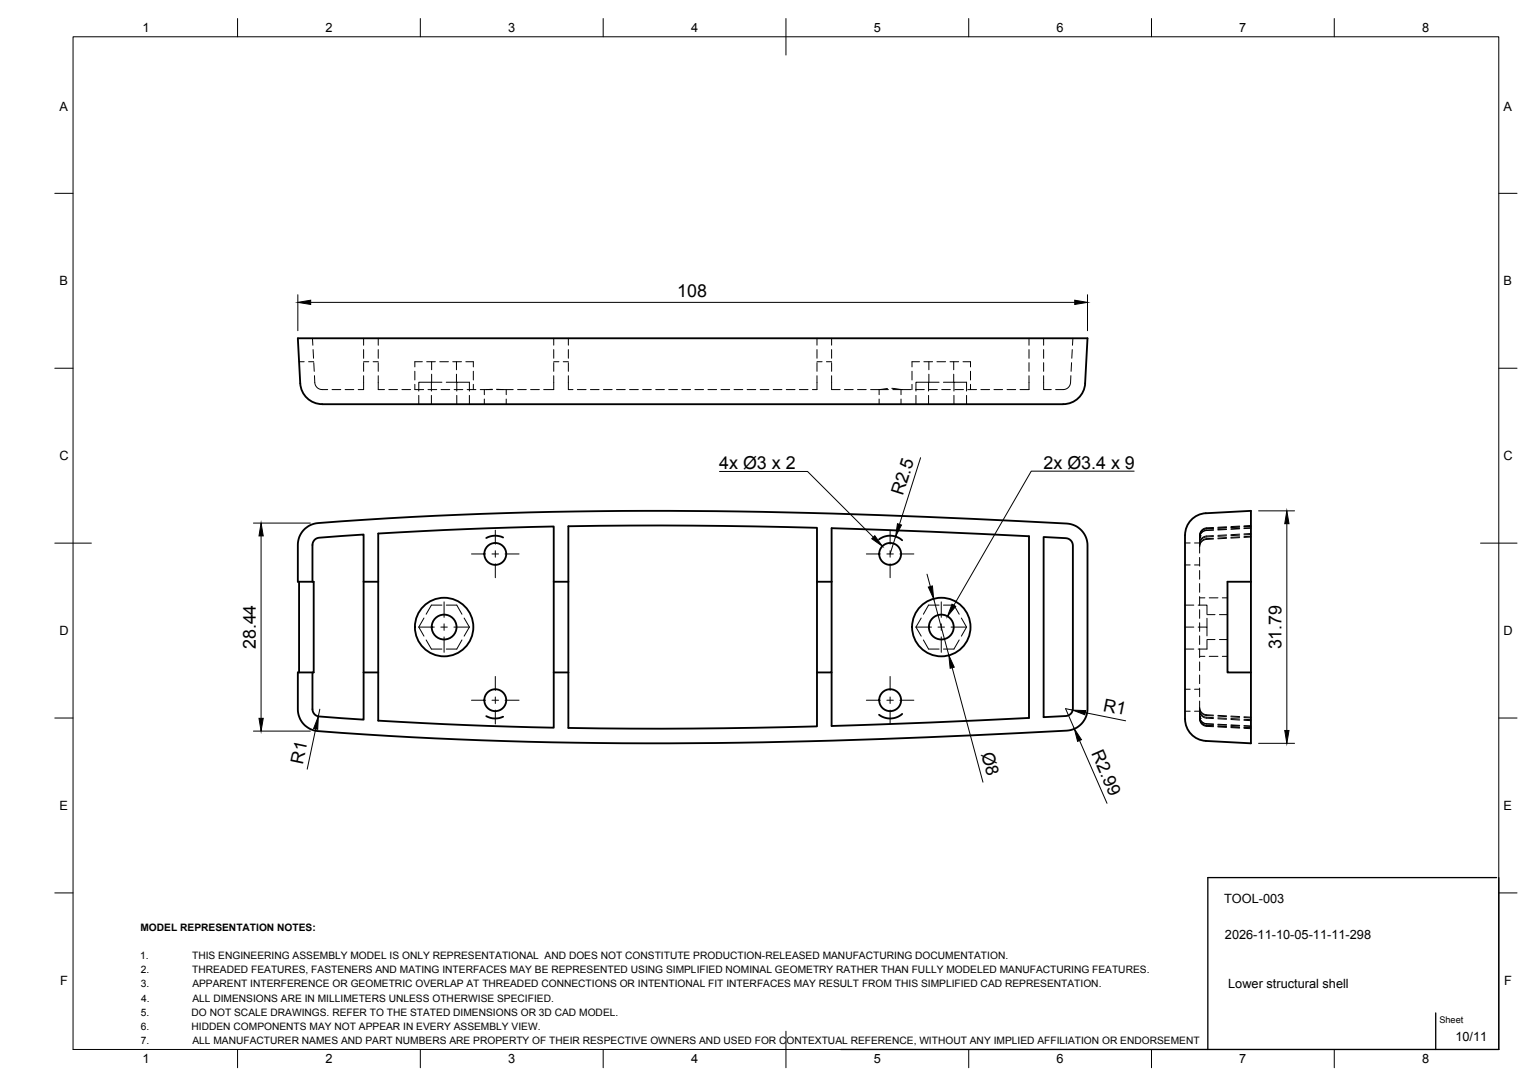
ISO-10303-21;
HEADER;
/* Generated by software containing ST-Developer
 * from STEP Tools, Inc. (www.steptools.com) 
 */

FILE_DESCRIPTION(
/* description */ (''),
/* implementation_level */ '2;1');

FILE_NAME(
/* name */ 'Lower structural shell.step',
/* time_stamp */ '2026-11-10T05:20:16-08:00',
/* author */ (''),
/* organization */ (''),
/* preprocessor_version */ 'ST-DEVELOPER v20.2',
/* originating_system */ 'Autodesk Translation Framework v15.17.0.0',
/* authorisation */ '');

FILE_SCHEMA (('AUTOMOTIVE_DESIGN { 1 0 10303 214 3 1 1 }'));
ENDSEC;

DATA;
#10=MECHANICAL_DESIGN_GEOMETRIC_PRESENTATION_REPRESENTATION('',(#117),#24809);
#84=SPHERICAL_SURFACE('',#10450,0.1);
#85=SPHERICAL_SURFACE('',#10453,0.0999999999999998);
#86=SPHERICAL_SURFACE('',#10457,0.0999999999999993);
#87=SPHERICAL_SURFACE('',#10461,0.1);
#88=SPHERICAL_SURFACE('',#10466,0.3);
#89=SPHERICAL_SURFACE('',#10470,0.3);
#90=SPHERICAL_SURFACE('',#10474,0.299999999999999);
#91=SPHERICAL_SURFACE('',#10479,0.3);
#97=SHAPE_REPRESENTATION_RELATIONSHIP('SRR','None',#24861,#107);
#107=ADVANCED_BREP_SHAPE_REPRESENTATION('',(#127),#24804);
#117=STYLED_ITEM('',(#24922),#127);
#127=MANIFOLD_SOLID_BREP('Body1',#9894);
#164=FACE_BOUND('',#2214,.T.);
#165=FACE_BOUND('',#2215,.T.);
#166=FACE_BOUND('',#2216,.T.);
#167=FACE_BOUND('',#2224,.T.);
#168=FACE_BOUND('',#2232,.T.);
#169=FACE_BOUND('',#2247,.T.);
#170=FACE_BOUND('',#2249,.T.);
#171=FACE_BOUND('',#2261,.T.);
#172=FACE_BOUND('',#2282,.T.);
#173=FACE_BOUND('',#2283,.T.);
#174=FACE_BOUND('',#2284,.T.);
#175=FACE_BOUND('',#2319,.T.);
#176=FACE_BOUND('',#2320,.T.);
#177=FACE_BOUND('',#2321,.T.);
#178=FACE_BOUND('',#2322,.T.);
#179=FACE_BOUND('',#2323,.T.);
#180=FACE_BOUND('',#2324,.T.);
#237=B_SPLINE_SURFACE_WITH_KNOTS('',3,3,((#17088,#17089,#17090,#17091),
(#17092,#17093,#17094,#17095),(#17096,#17097,#17098,#17099),(#17100,#17101,
#17102,#17103),(#17104,#17105,#17106,#17107)),.UNSPECIFIED.,.F.,.F.,.F.,
(4,1,4),(4,4),(0.,0.571428571428571,1.),(1.0454440030657,3.44967454744645),
 .UNSPECIFIED.);
#238=B_SPLINE_SURFACE_WITH_KNOTS('',3,3,((#17180,#17181,#17182,#17183),
(#17184,#17185,#17186,#17187),(#17188,#17189,#17190,#17191),(#17192,#17193,
#17194,#17195),(#17196,#17197,#17198,#17199)),.UNSPECIFIED.,.F.,.F.,.F.,
(4,1,4),(4,4),(0.,0.571428571428571,1.),(7.24519303641511,9.95046872158573),
 .UNSPECIFIED.);
#239=B_SPLINE_SURFACE_WITH_KNOTS('',3,3,((#18121,#18122,#18123,#18124),
(#18125,#18126,#18127,#18128),(#18129,#18130,#18131,#18132),(#18133,#18134,
#18135,#18136)),.UNSPECIFIED.,.F.,.F.,.F.,(4,4),(4,4),(0.0705535719740953,
0.323522444336189),(0.0117434863834119,0.684857763552191),.UNSPECIFIED.);
#240=B_SPLINE_SURFACE_WITH_KNOTS('',3,3,((#18141,#18142,#18143,#18144),
(#18145,#18146,#18147,#18148),(#18149,#18150,#18151,#18152),(#18153,#18154,
#18155,#18156)),.UNSPECIFIED.,.F.,.F.,.F.,(4,4),(4,4),(0.0262419052680539,
0.0545428296147404),(0.0121538053864343,0.684980602226481),
 .UNSPECIFIED.);
#241=B_SPLINE_SURFACE_WITH_KNOTS('',3,3,((#18166,#18167,#18168,#18169),
(#18170,#18171,#18172,#18173),(#18174,#18175,#18176,#18177),(#18178,#18179,
#18180,#18181),(#18182,#18183,#18184,#18185)),.UNSPECIFIED.,.F.,.F.,.F.,
(4,1,4),(4,4),(0.,0.571428571428571,1.),(0.752061768057538,3.45733745322815),
 .UNSPECIFIED.);
#242=B_SPLINE_SURFACE_WITH_KNOTS('',3,3,((#18186,#18187,#18188,#18189),
(#18190,#18191,#18192,#18193),(#18194,#18195,#18196,#18197),(#18198,#18199,
#18200,#18201),(#18202,#18203,#18204,#18205)),.UNSPECIFIED.,.F.,.F.,.F.,
(4,1,4),(4,4),(0.,0.571428571428571,1.),(0.283259008618247,0.557056952888827),
 .UNSPECIFIED.);
#243=B_SPLINE_SURFACE_WITH_KNOTS('',3,3,((#18219,#18220,#18221,#18222),
(#18223,#18224,#18225,#18226),(#18227,#18228,#18229,#18230),(#18231,#18232,
#18233,#18234)),.UNSPECIFIED.,.F.,.F.,.F.,(4,4),(4,4),(0.67647755566375,
0.929446428026011),(0.0117434863436937,0.684857763580381),.UNSPECIFIED.);
#244=B_SPLINE_SURFACE_WITH_KNOTS('',3,3,((#18235,#18236,#18237,#18238),
(#18239,#18240,#18241,#18242),(#18243,#18244,#18245,#18246),(#18247,#18248,
#18249,#18250)),.UNSPECIFIED.,.F.,.F.,.F.,(4,4),(4,4),(0.945457170385156,
0.973758094731946),(0.0121538053598088,0.684980602226481),.UNSPECIFIED.);
#245=B_SPLINE_SURFACE_WITH_KNOTS('',3,3,((#18334,#18335,#18336,#18337),
(#18338,#18339,#18340,#18341),(#18342,#18343,#18344,#18345),(#18346,#18347,
#18348,#18349)),.UNSPECIFIED.,.F.,.F.,.F.,(4,4),(4,4),(0.341142793678372,
0.658675488550287),(0.0116221239297273,0.684255166525269),.UNSPECIFIED.);
#246=B_SPLINE_SURFACE_WITH_KNOTS('',3,3,((#18354,#18355,#18356,#18357),
(#18358,#18359,#18360,#18361),(#18362,#18363,#18364,#18365),(#18366,#18367,
#18368,#18369),(#18370,#18371,#18372,#18373)),.UNSPECIFIED.,.F.,.F.,.F.,
(4,1,4),(4,4),(0.,0.571428571428571,1.),(3.65450559744172,7.0548588409572),
 .UNSPECIFIED.);
#247=B_SPLINE_SURFACE_WITH_KNOTS('',3,3,((#18383,#18384,#18385,#18386),
(#18387,#18388,#18389,#18390),(#18391,#18392,#18393,#18394),(#18395,#18396,
#18397,#18398),(#18399,#18400,#18401,#18402)),.UNSPECIFIED.,.F.,.F.,.F.,
(4,1,4),(4,4),(0.,0.571428571428571,1.),(3.64767164868607,7.04802489220155),
 .UNSPECIFIED.);
#248=B_SPLINE_SURFACE_WITH_KNOTS('',3,3,((#18407,#18408,#18409,#18410),
(#18411,#18412,#18413,#18414),(#18415,#18416,#18417,#18418),(#18419,#18420,
#18421,#18422)),.UNSPECIFIED.,.F.,.F.,.F.,(4,4),(4,4),(0.341324511449716,
0.658857206321627),(0.0116221214776208,0.684255166525269),.UNSPECIFIED.);
#249=B_SPLINE_SURFACE_WITH_KNOTS('',3,3,((#18467,#18468,#18469,#18470),
(#18471,#18472,#18473,#18474),(#18475,#18476,#18477,#18478),(#18479,#18480,
#18481,#18482)),.UNSPECIFIED.,.F.,.F.,.F.,(4,4),(4,4),(0.676316266718331,
0.901708040522105),(0.0117102006467275,0.68495201331719),.UNSPECIFIED.);
#250=B_SPLINE_SURFACE_WITH_KNOTS('',3,3,((#18487,#18488,#18489,#18490),
(#18491,#18492,#18493,#18494),(#18495,#18496,#18497,#18498),(#18499,#18500,
#18501,#18502),(#18503,#18504,#18505,#18506)),.UNSPECIFIED.,.F.,.F.,.F.,
(4,1,4),(4,4),(0.,0.571428571428571,1.),(7.25285594219682,9.65708648657758),
 .UNSPECIFIED.);
#251=B_SPLINE_SURFACE_WITH_KNOTS('',3,3,((#18516,#18517,#18518,#18519),
(#18520,#18521,#18522,#18523),(#18524,#18525,#18526,#18527),(#18528,#18529,
#18530,#18531)),.UNSPECIFIED.,.F.,.F.,.F.,(4,4),(4,4),(0.0982919594778951,
0.323683733281714),(0.0117102006467272,0.68495201331719),.UNSPECIFIED.);
#252=B_SPLINE_SURFACE_WITH_KNOTS('',3,3,((#18606,#18607,#18608,#18609),
(#18610,#18611,#18612,#18613),(#18614,#18615,#18616,#18617),(#18618,#18619,
#18620,#18621)),.UNSPECIFIED.,.F.,.F.,.F.,(4,4),(4,4),(0.917922863855343,
0.974411608827007),(0.0122403473423911,0.685344304754238),.UNSPECIFIED.);
#253=B_SPLINE_SURFACE_WITH_KNOTS('',3,3,((#18631,#18632,#18633,#18634),
(#18635,#18636,#18637,#18638),(#18639,#18640,#18641,#18642),(#18643,#18644,
#18645,#18646),(#18647,#18648,#18649,#18650)),.UNSPECIFIED.,.F.,.F.,.F.,
(4,1,4),(4,4),(0.,0.571428571428571,1.),(9.85085636625011,10.4271318523291),
 .UNSPECIFIED.);
#254=B_SPLINE_SURFACE_WITH_KNOTS('',3,3,((#18664,#18665,#18666,#18667),
(#18668,#18669,#18670,#18671),(#18672,#18673,#18674,#18675),(#18676,#18677,
#18678,#18679)),.UNSPECIFIED.,.F.,.F.,.F.,(4,4),(4,4),(0.025588391172993,
0.0820771361446569),(0.0122403473423911,0.685344304754238),
 .UNSPECIFIED.);
#255=B_SPLINE_SURFACE_WITH_KNOTS('',3,3,((#18689,#18690,#18691,#18692),
(#18693,#18694,#18695,#18696),(#18697,#18698,#18699,#18700),(#18701,#18702,
#18703,#18704),(#18705,#18706,#18707,#18708)),.UNSPECIFIED.,.F.,.F.,.F.,
(4,1,4),(4,4),(0.,0.571428571428571,1.),(0.27539863731415,0.851674123393175),
 .UNSPECIFIED.);
#256=B_SPLINE_SURFACE_WITH_KNOTS('',3,3,((#18722,#18723,#18724,#18725),
(#18726,#18727,#18728,#18729),(#18730,#18731,#18732,#18733),(#18734,#18735,
#18736,#18737),(#18738,#18739,#18740,#18741)),.UNSPECIFIED.,.F.,.F.,.F.,
(4,1,4),(4,4),(0.,0.571428571428571,1.),(0.00944995813270487,0.618489359031386),
 .UNSPECIFIED.);
#257=B_SPLINE_SURFACE_WITH_KNOTS('',3,3,((#18748,#18749,#18750,#18751),
(#18752,#18753,#18754,#18755),(#18756,#18757,#18758,#18759),(#18760,#18761,
#18762,#18763),(#18764,#18765,#18766,#18767)),.UNSPECIFIED.,.F.,.F.,.F.,
(4,1,4),(4,4),(0.,0.571428571428571,1.),(0.00908570715245136,0.618164468641375),
 .UNSPECIFIED.);
#258=B_SPLINE_SURFACE_WITH_KNOTS('',3,3,((#18772,#18773,#18774,#18775),
(#18776,#18777,#18778,#18779),(#18780,#18781,#18782,#18783),(#18784,#18785,
#18786,#18787),(#18788,#18789,#18790,#18791)),.UNSPECIFIED.,.F.,.F.,.F.,
(4,1,4),(4,4),(0.,0.571428571428571,1.),(0.0091183540525243,0.618164468641375),
 .UNSPECIFIED.);
#259=B_SPLINE_SURFACE_WITH_KNOTS('',3,3,((#18796,#18797,#18798,#18799),
(#18800,#18801,#18802,#18803),(#18804,#18805,#18806,#18807),(#18808,#18809,
#18810,#18811),(#18812,#18813,#18814,#18815)),.UNSPECIFIED.,.F.,.F.,.F.,
(4,1,4),(4,4),(0.,0.571428571428571,1.),(10.1454735367545,10.419271481025),
 .UNSPECIFIED.);
#260=B_SPLINE_SURFACE_WITH_KNOTS('',3,3,((#18816,#18817,#18818,#18819),
(#18820,#18821,#18822,#18823),(#18824,#18825,#18826,#18827),(#18828,#18829,
#18830,#18831),(#18832,#18833,#18834,#18835)),.UNSPECIFIED.,.F.,.F.,.F.,
(4,1,4),(4,4),(0.,0.571428571428571,1.),(0.0094045468285345,0.618489359031386),
 .UNSPECIFIED.);
#261=B_SPLINE_SURFACE_WITH_KNOTS('',3,3,((#18861,#18862,#18863,#18864),
(#18865,#18866,#18867,#18868),(#18869,#18870,#18871,#18872),(#18873,#18874,
#18875,#18876),(#18877,#18878,#18879,#18880)),.UNSPECIFIED.,.F.,.F.,.F.,
(4,1,4),(4,4),(0.,0.571428571428571,1.),(-0.00535061636073277,0.618489359031386),
 .UNSPECIFIED.);
#262=B_SPLINE_SURFACE_WITH_KNOTS('',3,3,((#18899,#18900,#18901,#18902,#18903),
(#18904,#18905,#18906,#18907,#18908),(#18909,#18910,#18911,#18912,#18913),
(#18914,#18915,#18916,#18917,#18918),(#18919,#18920,#18921,#18922,#18923)),
 .UNSPECIFIED.,.F.,.F.,.F.,(4,1,4),(4,1,4),(0.,0.571428571428571,1.),(0.283259008618247,
4.63063308449434,10.4271318523291),.UNSPECIFIED.);
#263=B_SPLINE_SURFACE_WITH_KNOTS('',3,3,((#18934,#18935,#18936,#18937),
(#18938,#18939,#18940,#18941),(#18942,#18943,#18944,#18945),(#18946,#18947,
#18948,#18949),(#18950,#18951,#18952,#18953)),.UNSPECIFIED.,.F.,.F.,.F.,
(4,1,4),(4,4),(0.,0.571428571428571,1.),(-0.00578978989683084,0.618164468641375),
 .UNSPECIFIED.);
#264=B_SPLINE_SURFACE_WITH_KNOTS('',3,3,((#18962,#18963,#18964,#18965),
(#18966,#18967,#18968,#18969),(#18970,#18971,#18972,#18973),(#18974,#18975,
#18976,#18977),(#18978,#18979,#18980,#18981)),.UNSPECIFIED.,.F.,.F.,.F.,
(4,1,4),(4,4),(0.,0.571428571428571,1.),(-0.00569189159989896,0.618164468641375),
 .UNSPECIFIED.);
#265=B_SPLINE_SURFACE_WITH_KNOTS('',3,3,((#18990,#18991,#18992,#18993,#18994),
(#18995,#18996,#18997,#18998,#18999),(#19000,#19001,#19002,#19003,#19004),
(#19005,#19006,#19007,#19008,#19009),(#19010,#19011,#19012,#19013,#19014)),
 .UNSPECIFIED.,.F.,.F.,.F.,(4,1,4),(4,1,4),(0.,0.571428571428571,1.),(0.27539863731415,
4.62277271319024,10.419271481025),.UNSPECIFIED.);
#266=B_SPLINE_SURFACE_WITH_KNOTS('',3,3,((#19025,#19026,#19027,#19028),
(#19029,#19030,#19031,#19032),(#19033,#19034,#19035,#19036),(#19037,#19038,
#19039,#19040),(#19041,#19042,#19043,#19044)),.UNSPECIFIED.,.F.,.F.,.F.,
(4,1,4),(4,4),(0.,0.571428571428571,1.),(-0.0054868135546625,0.618489359031386),
 .UNSPECIFIED.);
#267=B_SPLINE_SURFACE_WITH_KNOTS('',3,3,((#19053,#19054,#19055,#19056),
(#19057,#19058,#19059,#19060),(#19061,#19062,#19063,#19064),(#19065,#19066,
#19067,#19068)),.UNSPECIFIED.,.F.,.F.,.F.,(4,4),(4,4),(0.026239262514127,
0.974414173651419),(0.,0.685344304754238),.UNSPECIFIED.);
#268=B_SPLINE_SURFACE_WITH_KNOTS('',3,3,((#19071,#19072,#19073,#19074),
(#19075,#19076,#19077,#19078),(#19079,#19080,#19081,#19082),(#19083,#19084,
#19085,#19086)),.UNSPECIFIED.,.F.,.F.,.F.,(4,4),(4,4),(0.0255858263485814,
0.973760737485873),(0.,0.685344304754238),.UNSPECIFIED.);
#717=B_SPLINE_CURVE_WITH_KNOTS('',3,(#16987,#16988,#16989,#16990,#16991,
#16992,#16993,#16994,#16995,#16996,#16997,#16998,#16999,#17000,#17001,#17002,
#17003,#17004,#17005,#17006,#17007,#17008,#17009,#17010),.UNSPECIFIED.,
 .F.,.F.,(4,2,2,2,2,2,2,2,2,2,2,4),(-0.337265338267783,-0.250544943628509,
-0.208272806508042,-0.186542211788094,-0.176382978682897,-0.170925844043069,
-0.16639450677335,-0.161077381235501,-0.15182241135393,-0.115009181549223,
-0.030206004227969,0.),.UNSPECIFIED.);
#718=B_SPLINE_CURVE_WITH_KNOTS('',3,(#17015,#17016,#17017,#17018,#17019,
#17020,#17021,#17022,#17023,#17024,#17025,#17026,#17027,#17028,#17029,#17030,
#17031,#17032,#17033,#17034),.UNSPECIFIED.,.F.,.F.,(4,2,2,2,2,2,2,2,2,4),
(-0.240982594686416,-0.16829976149504,-0.141836598208813,-0.129116059226128,
-0.121962912034391,-0.115857591426886,-0.108506552485159,-0.0948769875819265,
-0.0364654790774683,0.),.UNSPECIFIED.);
#719=B_SPLINE_CURVE_WITH_KNOTS('',3,(#17039,#17040,#17041,#17042,#17043,
#17044,#17045,#17046,#17047,#17048,#17049,#17050,#17051,#17052,#17053,#17054,
#17055,#17056,#17057,#17058),.UNSPECIFIED.,.F.,.F.,(4,2,2,2,2,2,2,2,2,4),
(-0.240981214998207,-0.168303541671295,-0.141841407502325,-0.129121097580905,
-0.121968013294536,-0.115862708924237,-0.108511643765797,-0.0948818976588229,
-0.0364681276985956,0.),.UNSPECIFIED.);
#720=B_SPLINE_CURVE_WITH_KNOTS('',3,(#17063,#17064,#17065,#17066,#17067,
#17068,#17069,#17070,#17071,#17072,#17073,#17074,#17075,#17076,#17077,#17078,
#17079,#17080,#17081,#17082,#17083,#17084,#17085,#17086),.UNSPECIFIED.,
 .F.,.F.,(4,2,2,2,2,2,2,2,2,2,2,4),(-0.337269388373684,-0.250545316912909,
-0.208282401844766,-0.186554569827561,-0.176396213396297,-0.17093921790305,
-0.16640782243471,-0.161090427650893,-0.151834477986603,-0.115010808423941,
-0.0302102096065556,0.),.UNSPECIFIED.);
#721=B_SPLINE_CURVE_WITH_KNOTS('',3,(#17109,#17110,#17111,#17112),
 .UNSPECIFIED.,.F.,.F.,(4,4),(1.0454440030657,2.52465537163019),
 .UNSPECIFIED.);
#722=B_SPLINE_CURVE_WITH_KNOTS('',3,(#17114,#17115,#17116,#17117,#17118,
#17119,#17120,#17121,#17122,#17123,#17124,#17125,#17126,#17127,#17128,#17129,
#17130,#17131,#17132,#17133,#17134,#17135,#17136,#17137,#17138,#17139,#17140,
#17141),.UNSPECIFIED.,.F.,.F.,(4,3,3,3,3,3,3,3,3,4),(-0.152193408756968,
-0.128427023368412,-0.115107736263918,-0.0911810900745799,-0.0780377802127556,
-0.0652031397886901,-0.0414031558437525,-0.0389949527774582,-0.0152076153333754,
0.),.UNSPECIFIED.);
#723=B_SPLINE_CURVE_WITH_KNOTS('',3,(#17143,#17144,#17145,#17146),
 .UNSPECIFIED.,.F.,.F.,(4,4),(-3.44967454744645,-1.05170160817356),
 .UNSPECIFIED.);
#724=B_SPLINE_CURVE_WITH_KNOTS('',3,(#17148,#17149,#17150,#17151,#17152,
#17153,#17154,#17155,#17156,#17157,#17158,#17159,#17160,#17161,#17162,#17163,
#17164,#17165,#17166,#17167,#17168,#17169,#17170,#17171,#17172,#17173,#17174,
#17175),.UNSPECIFIED.,.F.,.F.,(4,3,3,3,3,3,3,3,3,4),(-0.152278960443096,
-0.128503570101575,-0.115218572146868,-0.09145408274965,-0.0870214650669139,
-0.0781562978024333,-0.0542566895399357,-0.03908030849237,-0.0153296112319379,
0.),.UNSPECIFIED.);
#725=B_SPLINE_CURVE_WITH_KNOTS('',3,(#17176,#17177,#17178,#17179),
 .UNSPECIFIED.,.F.,.F.,(4,4),(2.75501813708031,3.4476340663212),
 .UNSPECIFIED.);
#726=B_SPLINE_CURVE_WITH_KNOTS('',3,(#17201,#17202,#17203,#17204),
 .UNSPECIFIED.,.F.,.F.,(4,4),(7.24810383506675,7.89761558728778),
 .UNSPECIFIED.);
#727=B_SPLINE_CURVE_WITH_KNOTS('',3,(#17206,#17207,#17208,#17209,#17210,
#17211,#17212,#17213,#17214,#17215,#17216,#17217,#17218,#17219,#17220,#17221,
#17222,#17223,#17224,#17225,#17226,#17227,#17228,#17229,#17230,#17231,#17232,
#17233),.UNSPECIFIED.,.F.,.F.,(4,3,3,3,3,3,3,3,3,4),(-0.152278869104567,
-0.128548794904564,-0.115192257893812,-0.0912773536606376,-0.0781090575823055,
-0.0652724057916263,-0.0414819581560496,-0.0390493575290778,-0.015259721743698,
0.),.UNSPECIFIED.);
#728=B_SPLINE_CURVE_WITH_KNOTS('',3,(#17235,#17236,#17237,#17238),
 .UNSPECIFIED.,.F.,.F.,(4,4),(-9.94532343034734,-7.24519303641511),
 .UNSPECIFIED.);
#729=B_SPLINE_CURVE_WITH_KNOTS('',3,(#17240,#17241,#17242,#17243,#17244,
#17245,#17246,#17247,#17248,#17249,#17250,#17251,#17252,#17253,#17254,#17255,
#17256,#17257,#17258,#17259,#17260,#17261,#17262,#17263,#17264,#17265,#17266,
#17267),.UNSPECIFIED.,.F.,.F.,(4,3,3,3,3,3,3,3,3,4),(-0.152181623618259,
-0.128410404494075,-0.115248188224843,-0.0914746846046984,-0.0869904866333268,
-0.0783028696190655,-0.0543945376065823,-0.0391651209697638,-0.0153884182770307,
0.),.UNSPECIFIED.);
#730=B_SPLINE_CURVE_WITH_KNOTS('',3,(#17268,#17269,#17270,#17271),
 .UNSPECIFIED.,.F.,.F.,(4,4),(8.21380824320284,9.95046871680089),
 .UNSPECIFIED.);
#731=B_SPLINE_CURVE_WITH_KNOTS('',3,(#17274,#17275,#17276,#17277),
 .UNSPECIFIED.,.F.,.F.,(4,4),(2.80491490332713,3.45442665446657),
 .UNSPECIFIED.);
#732=B_SPLINE_CURVE_WITH_KNOTS('',3,(#17281,#17282,#17283,#17284),
 .UNSPECIFIED.,.F.,.F.,(4,4),(0.752061768057538,2.48872224644044),
 .UNSPECIFIED.);
#733=B_SPLINE_CURVE_WITH_KNOTS('',3,(#17492,#17493,#17494,#17495,#17496,
#17497),.UNSPECIFIED.,.F.,.F.,(4,2,4),(-0.606700505977711,-0.303383635264422,
-0.000339350725729326),.UNSPECIFIED.);
#734=B_SPLINE_CURVE_WITH_KNOTS('',3,(#17498,#17499,#17500,#17501,#17502,
#17503,#17504,#17505,#17506,#17507,#17508,#17509,#17510,#17511,#17512,#17513,
#17514,#17515,#17516,#17517,#17518,#17519,#17520,#17521,#17522,#17523,#17524,
#17525),.UNSPECIFIED.,.F.,.F.,(4,3,3,3,3,3,3,3,3,4),(-0.152173579228948,
-0.128423230539522,-0.115115104157663,-0.0911927259648815,-0.0780672068328041,
-0.0652082609452843,-0.0414117413801899,-0.0390174000215468,-0.0152300060615686,
0.),.UNSPECIFIED.);
#735=B_SPLINE_CURVE_WITH_KNOTS('',3,(#17526,#17527,#17528,#17529,#17530,
#17531),.UNSPECIFIED.,.F.,.F.,(4,2,4),(-0.606471894652381,-0.303383500305553,
-0.00011071898471493),.UNSPECIFIED.);
#736=B_SPLINE_CURVE_WITH_KNOTS('',3,(#17535,#17536,#17537,#17538,#17539,
#17540),.UNSPECIFIED.,.F.,.F.,(4,2,4),(-0.606240625011114,-0.303433113375332,
-0.00010938105916114),.UNSPECIFIED.);
#737=B_SPLINE_CURVE_WITH_KNOTS('',3,(#17542,#17543,#17544,#17545,#17546,
#17547,#17548,#17549,#17550,#17551,#17552,#17553,#17554,#17555,#17556,#17557,
#17558,#17559,#17560,#17561,#17562,#17563,#17564,#17565,#17566,#17567,#17568,
#17569),.UNSPECIFIED.,.F.,.F.,(4,3,3,3,3,3,3,3,3,4),(-0.152281454644235,
-0.128508102092242,-0.115234945630277,-0.0914677943501604,-0.0870276017853555,
-0.0781846052914712,-0.0542821334115454,-0.0390966859411886,-0.0153419673568312,
0.),.UNSPECIFIED.);
#738=B_SPLINE_CURVE_WITH_KNOTS('',3,(#17571,#17572,#17573,#17574,#17575,
#17576),.UNSPECIFIED.,.F.,.F.,(4,2,4),(-0.606758573154242,-0.303433157101101,
-0.000627306481538803),.UNSPECIFIED.);
#739=B_SPLINE_CURVE_WITH_KNOTS('',3,(#17582,#17583,#17584,#17585,#17586,
#17587),.UNSPECIFIED.,.F.,.F.,(4,2,4),(-0.60617382748,-0.303436117212405,
-7.2700296824213E-5),.UNSPECIFIED.);
#740=B_SPLINE_CURVE_WITH_KNOTS('',3,(#17589,#17590,#17591,#17592,#17593,
#17594,#17595,#17596,#17597,#17598,#17599,#17600,#17601,#17602,#17603,#17604,
#17605,#17606,#17607,#17608,#17609,#17610,#17611,#17612,#17613,#17614,#17615,
#17616),.UNSPECIFIED.,.F.,.F.,(4,3,3,3,3,3,3,3,3,4),(-0.152282154327755,
-0.128558036203745,-0.115201429639692,-0.0912891813973639,-0.0781219052297615,
-0.065279687589213,-0.0414913146723999,-0.0390591331507366,-0.0152683745546824,
0.),.UNSPECIFIED.);
#741=B_SPLINE_CURVE_WITH_KNOTS('',3,(#17620,#17621,#17622,#17623,#17624,
#17625,#17626,#17627,#17628,#17629,#17630,#17631,#17632,#17633,#17634,#17635,
#17636,#17637,#17638,#17639,#17640,#17641,#17642,#17643,#17644,#17645,#17646,
#17647),.UNSPECIFIED.,.F.,.F.,(4,3,3,3,3,3,3,3,3,4),(-0.152283066055976,
-0.128508717930245,-0.115216472798554,-0.091451700383826,-0.087022506454752,
-0.0781485278686168,-0.0542483994686567,-0.0390758108455304,-0.0153274175274101,
0.),.UNSPECIFIED.);
#742=B_SPLINE_CURVE_WITH_KNOTS('',3,(#17649,#17650,#17651,#17652,#17653,
#17654),.UNSPECIFIED.,.F.,.F.,(4,2,4),(-0.606800264911061,-0.303436147592132,
-0.000699137727853738),.UNSPECIFIED.);
#743=B_SPLINE_CURVE_WITH_KNOTS('',3,(#17659,#17660,#17661,#17662,#17663,
#17664),.UNSPECIFIED.,.F.,.F.,(4,2,4),(-0.606915279655722,-0.30363236403835,
-0.000516487074480598),.UNSPECIFIED.);
#744=B_SPLINE_CURVE_WITH_KNOTS('',3,(#17668,#17669,#17670,#17671,#17672,
#17673,#17674,#17675,#17676,#17677,#17678,#17679,#17680,#17681,#17682,#17683,
#17684,#17685,#17686,#17687,#17688,#17689,#17690,#17691,#17692,#17693,#17694,
#17695),.UNSPECIFIED.,.F.,.F.,(4,3,3,3,3,3,3,3,3,4),(-0.152205325335401,
-0.128433618138404,-0.115304790388008,-0.091527299141506,-0.0870178586418932,
-0.0783866443643876,-0.0544751548276533,-0.0392137310602028,-0.0154203878854647,
0.),.UNSPECIFIED.);
#745=B_SPLINE_CURVE_WITH_KNOTS('',3,(#17697,#17698,#17699,#17700,#17701,
#17702),.UNSPECIFIED.,.F.,.F.,(4,2,4),(-0.606752424187958,-0.303632696349781,
-0.000353591088346872),.UNSPECIFIED.);
#746=B_SPLINE_CURVE_WITH_KNOTS('',3,(#17708,#17709,#17710,#17711),
 .UNSPECIFIED.,.F.,.F.,(4,4),(0.0116023361771303,0.618489359031386),
 .UNSPECIFIED.);
#747=B_SPLINE_CURVE_WITH_KNOTS('',3,(#17715,#17716,#17717,#17718),
 .UNSPECIFIED.,.F.,.F.,(4,4),(-0.618489359031386,-0.01160233617713),
 .UNSPECIFIED.);
#748=B_SPLINE_CURVE_WITH_KNOTS('',3,(#17721,#17722,#17723,#17724),
 .UNSPECIFIED.,.F.,.F.,(4,4),(7.01593971618694,9.71770560667459),
 .UNSPECIFIED.);
#749=B_SPLINE_CURVE_WITH_KNOTS('',3,(#17725,#17726,#17727,#17728),
 .UNSPECIFIED.,.F.,.F.,(4,4),(0.505945342046796,3.20718651982575),
 .UNSPECIFIED.);
#750=B_SPLINE_CURVE_WITH_KNOTS('',3,(#17731,#17732,#17733,#17734,#17735,
#17736,#17737),.UNSPECIFIED.,.F.,.F.,(4,3,4),(3.40717417387402,5.11170895874517,
6.80746068626633),.UNSPECIFIED.);
#751=B_SPLINE_CURVE_WITH_KNOTS('',3,(#17740,#17741,#17742,#17743),
 .UNSPECIFIED.,.F.,.F.,(4,4),(7.00766573366377,9.41198845520559),
 .UNSPECIFIED.);
#752=B_SPLINE_CURVE_WITH_KNOTS('',3,(#17747,#17748,#17749,#17750),
 .UNSPECIFIED.,.F.,.F.,(4,4),(9.61248784142317,10.2217363065808),
 .UNSPECIFIED.);
#753=B_SPLINE_CURVE_WITH_KNOTS('',3,(#17751,#17752,#17753,#17754,#17755,
#17756,#17757,#17758,#17759,#17760,#17761,#17762,#17763,#17764,#17765,#17766,
#17767,#17768,#17769,#17770,#17771,#17772,#17773,#17774,#17775,#17776,#17777,
#17778),.UNSPECIFIED.,.F.,.F.,(4,3,3,3,3,3,3,3,3,4),(0.,0.0238103109064959,
0.0390781362249314,0.0628635086275546,0.0641230352384255,0.0780643700703951,
0.101962174814111,0.113803522271848,0.137549611554782,0.149564734365165),
 .UNSPECIFIED.);
#754=B_SPLINE_CURVE_WITH_KNOTS('',3,(#17782,#17783,#17784,#17785,#17786,
#17787,#17788,#17789,#17790,#17791,#17792,#17793,#17794,#17795,#17796,#17797,
#17798,#17799,#17800,#17801,#17802,#17803,#17804,#17805,#17806,#17807,#17808,
#17809,#17810,#17811,#17812),.UNSPECIFIED.,.F.,.F.,(4,3,3,3,3,3,3,3,3,3,
4),(0.,0.0535521515156599,0.107729685495911,0.117233338918226,0.171447998942947,
0.1923696899792,0.234191611538245,0.288659693466396,0.341410301570312,0.395549383747909,
0.448696573746633),.UNSPECIFIED.);
#755=B_SPLINE_CURVE_WITH_KNOTS('',3,(#17814,#17815,#17816,#17817),
 .UNSPECIFIED.,.F.,.F.,(4,4),(0.0255858263485814,0.973760737485873),
 .UNSPECIFIED.);
#756=B_SPLINE_CURVE_WITH_KNOTS('',3,(#17819,#17820,#17821,#17822,#17823,
#17824,#17825,#17826,#17827,#17828,#17829,#17830,#17831,#17832,#17833,#17834,
#17835,#17836,#17837,#17838,#17839,#17840,#17841,#17842,#17843,#17844,#17845,
#17846,#17847,#17848,#17849),.UNSPECIFIED.,.F.,.F.,(4,3,3,3,3,3,3,3,3,3,
4),(0.,0.0535144560117858,0.107726856902975,0.117300577410231,0.171517675930231,
0.195438847090422,0.234297456941738,0.289665153342662,0.345032849743585,
0.40043206955427,0.455831289364955),.UNSPECIFIED.);
#757=B_SPLINE_CURVE_WITH_KNOTS('',3,(#17853,#17854,#17855,#17856,#17857,
#17858,#17859,#17860,#17861,#17862,#17863,#17864,#17865,#17866,#17867,#17868,
#17869,#17870,#17871,#17872,#17873,#17874,#17875,#17876,#17877,#17878,#17879,
#17880,#17881,#17882,#17883),.UNSPECIFIED.,.F.,.F.,(4,3,3,3,3,3,3,3,3,3,
4),(0.,0.053505543180391,0.107714168832353,0.117253997025819,0.171473395203321,
0.195418854185489,0.234223199196375,0.289607016015183,0.344990832833991,
0.400409777473312,0.455828722112633),.UNSPECIFIED.);
#758=B_SPLINE_CURVE_WITH_KNOTS('',3,(#17885,#17886,#17887,#17888),
 .UNSPECIFIED.,.F.,.F.,(4,4),(0.0262392625141271,0.974414173651419),
 .UNSPECIFIED.);
#759=B_SPLINE_CURVE_WITH_KNOTS('',3,(#17890,#17891,#17892,#17893,#17894,
#17895,#17896,#17897,#17898,#17899,#17900,#17901,#17902,#17903,#17904,#17905,
#17906,#17907,#17908,#17909,#17910,#17911,#17912,#17913,#17914,#17915,#17916,
#17917,#17918,#17919,#17920),.UNSPECIFIED.,.F.,.F.,(4,3,3,3,3,3,3,3,3,3,
4),(0.,0.0535648734523888,0.107747221190676,0.117299947751206,0.171510987106922,
0.192397607227928,0.234296687348373,0.288768001369001,0.341469499352622,
0.395597672314973,0.448700135162036),.UNSPECIFIED.);
#760=B_SPLINE_CURVE_WITH_KNOTS('',3,(#17923,#17924,#17925,#17926,#17927,
#17928,#17929,#17930,#17931,#17932,#17933,#17934,#17935,#17936,#17937,#17938,
#17939,#17940,#17941,#17942,#17943,#17944,#17945,#17946,#17947),
 .UNSPECIFIED.,.F.,.F.,(4,3,3,3,3,3,3,3,4),(0.,0.0238141989470671,0.0391004231578824,
0.0641320992313133,0.0780996136084711,0.101998806889826,0.113823260594808,
0.137564745199532,0.149565921982294),.UNSPECIFIED.);
#761=B_SPLINE_CURVE_WITH_KNOTS('',3,(#17949,#17950,#17951,#17952),
 .UNSPECIFIED.,.F.,.F.,(4,4),(2.76692059912875E-5,0.609394470571143),
 .UNSPECIFIED.);
#762=B_SPLINE_CURVE_WITH_KNOTS('',3,(#17955,#17956,#17957,#17958),
 .UNSPECIFIED.,.F.,.F.,(4,4),(0.809932799154201,3.21472245120952),
 .UNSPECIFIED.);
#763=B_SPLINE_CURVE_WITH_KNOTS('',3,(#17961,#17962,#17963,#17964,#17965,
#17966,#17967),.UNSPECIFIED.,.F.,.F.,(4,3,4),(3.41496637450242,5.11093193409745,
6.81591321610411),.UNSPECIFIED.);
#764=B_SPLINE_CURVE_WITH_KNOTS('',3,(#17971,#17972,#17973,#17974),
 .UNSPECIFIED.,.F.,.F.,(4,4),(9.91798263530139,10.2237206759544),
 .UNSPECIFIED.);
#765=B_SPLINE_CURVE_WITH_KNOTS('',3,(#17976,#17977,#17978,#17979,#17980,
#17981,#17982,#17983,#17984,#17985,#17986,#17987,#17988,#17989,#17990,#17991,
#17992,#17993,#17994,#17995,#17996,#17997,#17998,#17999,#18000,#18001,#18002,
#18003),.UNSPECIFIED.,.F.,.F.,(4,3,3,3,3,3,3,3,3,4),(0.,0.023807020713713,
0.039085080816122,0.0628703378723092,0.0651394887354207,0.0780750047750988,
0.101981498769656,0.114997221725907,0.138748569029605,0.151942344104828),
 .UNSPECIFIED.);
#766=B_SPLINE_CURVE_WITH_KNOTS('',3,(#18007,#18008,#18009,#18010,#18011,
#18012,#18013,#18014,#18015,#18016,#18017,#18018,#18019,#18020,#18021,#18022,
#18023,#18024,#18025,#18026,#18027,#18028,#18029,#18030,#18031,#18032,#18033,
#18034),.UNSPECIFIED.,.F.,.F.,(4,3,3,3,3,3,3,3,3,4),(0.,0.0238098191818892,
0.0391006681981376,0.0628849269680955,0.0651459659463291,0.0780999162396042,
0.102007524384594,0.115011225379555,0.138759376430353,0.151943200125079),
 .UNSPECIFIED.);
#767=B_SPLINE_CURVE_WITH_KNOTS('',3,(#18036,#18037,#18038,#18039),
 .UNSPECIFIED.,.F.,.F.,(4,4),(2.85486020485948E-5,0.305707210239178),
 .UNSPECIFIED.);
#768=B_SPLINE_CURVE_WITH_KNOTS('',3,(#18049,#18050,#18051,#18052,#18053,
#18054),.UNSPECIFIED.,.F.,.F.,(4,2,4),(-0.606446248197249,-0.303383959626182,
-6.4365448350312E-5),.UNSPECIFIED.);
#769=B_SPLINE_CURVE_WITH_KNOTS('',3,(#18056,#18057,#18058,#18059,#18060,
#18061),.UNSPECIFIED.,.F.,.F.,(4,2,4),(-0.60675170080159,-0.303384112192838,
-0.000369837888147484),.UNSPECIFIED.);
#770=B_SPLINE_CURVE_WITH_KNOTS('',3,(#18063,#18064,#18065,#18066,#18067,
#18068,#18069,#18070,#18071,#18072,#18073,#18074,#18075,#18076,#18077,#18078,
#18079,#18080,#18081,#18082,#18083,#18084,#18085,#18086,#18087,#18088,#18089,
#18090),.UNSPECIFIED.,.F.,.F.,(4,3,3,3,3,3,3,3,3,4),(-0.152162866344201,
-0.128411131698784,-0.115108013904405,-0.0911850729173883,-0.0780642464630149,
-0.0652023242402653,-0.0414053499882389,-0.0390151293250392,-0.0152279490549848,
0.),.UNSPECIFIED.);
#771=B_SPLINE_CURVE_WITH_KNOTS('',3,(#18093,#18094,#18095,#18096,#18097,
#18098,#18099,#18100,#18101,#18102,#18103,#18104,#18105,#18106,#18107,#18108,
#18109,#18110,#18111,#18112,#18113,#18114,#18115,#18116,#18117,#18118,#18119,
#18120),.UNSPECIFIED.,.F.,.F.,(4,3,3,3,3,3,3,3,3,4),(-0.152171297476962,
-0.128400300768352,-0.115247520946962,-0.0914735511738372,-0.0869860114952295,
-0.0783112904282795,-0.0544025203706761,-0.0391699941254272,-0.015391764586027,
0.),.UNSPECIFIED.);
#772=B_SPLINE_CURVE_WITH_KNOTS('',3,(#18137,#18138,#18139,#18140),
 .UNSPECIFIED.,.F.,.F.,(4,4),(-3.45733745322815,-0.757207059295936),
 .UNSPECIFIED.);
#773=B_SPLINE_CURVE_WITH_KNOTS('',3,(#18158,#18159,#18160,#18161),
 .UNSPECIFIED.,.F.,.F.,(4,4),(-0.557056952888827,-0.283259008618247),
 .UNSPECIFIED.);
#774=B_SPLINE_CURVE_WITH_KNOTS('',3,(#18162,#18163,#18164,#18165),
 .UNSPECIFIED.,.F.,.F.,(4,4),(-0.618164468641375,-0.0110156167597059),
 .UNSPECIFIED.);
#775=B_SPLINE_CURVE_WITH_KNOTS('',3,(#18207,#18208,#18209,#18210),
 .UNSPECIFIED.,.F.,.F.,(4,4),(0.283259011433088,0.551788488929761),
 .UNSPECIFIED.);
#776=B_SPLINE_CURVE_WITH_KNOTS('',3,(#18214,#18215,#18216,#18217),
 .UNSPECIFIED.,.F.,.F.,(4,4),(10.1507419987596,10.419271481025),
 .UNSPECIFIED.);
#777=B_SPLINE_CURVE_WITH_KNOTS('',3,(#18252,#18253,#18254,#18255),
 .UNSPECIFIED.,.F.,.F.,(4,4),(0.0110156167597055,0.618164468641375),
 .UNSPECIFIED.);
#778=B_SPLINE_CURVE_WITH_KNOTS('',3,(#18256,#18257,#18258,#18259),
 .UNSPECIFIED.,.F.,.F.,(4,4),(-10.419271481025,-10.1454735367545),
 .UNSPECIFIED.);
#779=B_SPLINE_CURVE_WITH_KNOTS('',3,(#18262,#18263,#18264,#18265,#18266,
#18267),.UNSPECIFIED.,.F.,.F.,(4,2,4),(-0.606211482799139,-0.303431960476852,
-9.19895310989571E-5),.UNSPECIFIED.);
#780=B_SPLINE_CURVE_WITH_KNOTS('',3,(#18269,#18270,#18271,#18272,#18273,
#18274,#18275,#18276,#18277,#18278,#18279,#18280,#18281,#18282,#18283,#18284,
#18285,#18286,#18287,#18288,#18289,#18290,#18291,#18292,#18293,#18294,#18295,
#18296),.UNSPECIFIED.,.F.,.F.,(4,3,3,3,3,3,3,3,3,4),(-0.152283340966725,
-0.128554242174982,-0.115196092098682,-0.0912819860997417,-0.0781117853096875,
-0.0652755629514801,-0.0414857317972147,-0.039051434275634,-0.0152612146291672,
0.),.UNSPECIFIED.);
#781=B_SPLINE_CURVE_WITH_KNOTS('',3,(#18300,#18301,#18302,#18303,#18304,
#18305,#18306,#18307,#18308,#18309,#18310,#18311,#18312,#18313,#18314,#18315,
#18316,#18317,#18318,#18319,#18320,#18321,#18322,#18323,#18324,#18325,#18326,
#18327),.UNSPECIFIED.,.F.,.F.,(4,3,3,3,3,3,3,3,3,4),(-0.152285570909379,
-0.128511627155755,-0.115232904621082,-0.0914664612111958,-0.0870286654075453,
-0.0781769338106538,-0.0542752301960614,-0.039092246575741,-0.0153386136911565,
0.),.UNSPECIFIED.);
#782=B_SPLINE_CURVE_WITH_KNOTS('',3,(#18328,#18329,#18330,#18331,#18332,
#18333),.UNSPECIFIED.,.F.,.F.,(4,2,4),(-0.606773318344362,-0.303431998667662,
-0.000653802131222458),.UNSPECIFIED.);
#783=B_SPLINE_CURVE_WITH_KNOTS('',3,(#18350,#18351,#18352,#18353),
 .UNSPECIFIED.,.F.,.F.,(4,4),(-7.05313168653828,-3.6572084986735),
 .UNSPECIFIED.);
#784=B_SPLINE_CURVE_WITH_KNOTS('',3,(#18374,#18375,#18376,#18377),
 .UNSPECIFIED.,.F.,.F.,(4,4),(3.65450559744172,7.0548588409572),
 .UNSPECIFIED.);
#785=B_SPLINE_CURVE_WITH_KNOTS('',3,(#18379,#18380,#18381,#18382),
 .UNSPECIFIED.,.F.,.F.,(4,4),(3.64767164868607,7.04802489220155),
 .UNSPECIFIED.);
#786=B_SPLINE_CURVE_WITH_KNOTS('',3,(#18403,#18404,#18405,#18406),
 .UNSPECIFIED.,.F.,.F.,(4,4),(-7.04532199096977,-3.64939880310499),
 .UNSPECIFIED.);
#787=B_SPLINE_CURVE_WITH_KNOTS('',3,(#18425,#18426,#18427,#18428,#18429,
#18430),.UNSPECIFIED.,.F.,.F.,(4,2,4),(-0.606200453641641,-0.30343602424441,
-9.0120313562092E-5),.UNSPECIFIED.);
#788=B_SPLINE_CURVE_WITH_KNOTS('',3,(#18432,#18433,#18434,#18435,#18436,
#18437,#18438,#18439,#18440,#18441,#18442,#18443,#18444,#18445,#18446,#18447,
#18448,#18449,#18450,#18451,#18452,#18453,#18454,#18455,#18456,#18457,#18458,
#18459),.UNSPECIFIED.,.F.,.F.,(4,3,3,3,3,3,3,3,3,4),(-0.152277688086818,
-0.128551334178815,-0.115197577176818,-0.0912856014461669,-0.0781191417238373,
-0.0652765169533013,-0.0414883027365163,-0.0390570310290822,-0.0152653090895913,
0.),.UNSPECIFIED.);
#789=B_SPLINE_CURVE_WITH_KNOTS('',3,(#18461,#18462,#18463,#18464,#18465,
#18466),.UNSPECIFIED.,.F.,.F.,(4,2,4),(-0.60678286609787,-0.303436074842897,
-0.000672492961417026),.UNSPECIFIED.);
#790=B_SPLINE_CURVE_WITH_KNOTS('',3,(#18483,#18484,#18485,#18486),
 .UNSPECIFIED.,.F.,.F.,(4,4),(-9.65082888146972,-7.25285594219682),
 .UNSPECIFIED.);
#791=B_SPLINE_CURVE_WITH_KNOTS('',3,(#18507,#18508,#18509,#18510),
 .UNSPECIFIED.,.F.,.F.,(4,4),(7.25489642332205,7.94751235889625),
 .UNSPECIFIED.);
#792=B_SPLINE_CURVE_WITH_KNOTS('',3,(#18511,#18512,#18513,#18514),
 .UNSPECIFIED.,.F.,.F.,(4,4),(8.17787511801303,9.65708648657758),
 .UNSPECIFIED.);
#793=B_SPLINE_CURVE_WITH_KNOTS('',3,(#18534,#18535,#18536,#18537,#18538,
#18539),.UNSPECIFIED.,.F.,.F.,(4,2,4),(-0.607007797795788,-0.303636495504298,
-0.000571323176327465),.UNSPECIFIED.);
#794=B_SPLINE_CURVE_WITH_KNOTS('',3,(#18541,#18542,#18543,#18544,#18545,
#18546,#18547,#18548,#18549,#18550,#18551,#18552,#18553,#18554,#18555,#18556,
#18557,#18558,#18559,#18560,#18561,#18562,#18563,#18564,#18565,#18566,#18567,
#18568),.UNSPECIFIED.,.F.,.F.,(4,3,3,3,3,3,3,3,3,4),(-0.152184339020145,
-0.128410461444444,-0.115096394428865,-0.0911692948751363,-0.0780261759644403,
-0.0651939085034322,-0.0413932235702045,-0.0389860720679279,-0.0151971168406065,
0.),.UNSPECIFIED.);
#795=B_SPLINE_CURVE_WITH_KNOTS('',3,(#18572,#18573,#18574,#18575,#18576,
#18577,#18578,#18579,#18580,#18581,#18582,#18583,#18584,#18585,#18586,#18587,
#18588,#18589,#18590,#18591,#18592,#18593,#18594,#18595,#18596,#18597,#18598,
#18599),.UNSPECIFIED.,.F.,.F.,(4,3,3,3,3,3,3,3,3,4),(-0.15219777746951,
-0.128424216118147,-0.115318679085322,-0.0915406112613293,-0.0870190514838729,
-0.0784197287877601,-0.0545085386658457,-0.0392329067084975,-0.0154317870320417,
0.),.UNSPECIFIED.);
#796=B_SPLINE_CURVE_WITH_KNOTS('',3,(#18600,#18601,#18602,#18603,#18604,
#18605),.UNSPECIFIED.,.F.,.F.,(4,2,4),(-0.606706256981509,-0.303636876939173,
-0.00026974181288697),.UNSPECIFIED.);
#797=B_SPLINE_CURVE_WITH_KNOTS('',3,(#18623,#18624,#18625,#18626),
 .UNSPECIFIED.,.F.,.F.,(4,4),(0.0112334529114386,0.618489359031386),
 .UNSPECIFIED.);
#798=B_SPLINE_CURVE_WITH_KNOTS('',3,(#18627,#18628,#18629,#18630),
 .UNSPECIFIED.,.F.,.F.,(4,4),(-10.4271318523291,-9.85085636625011),
 .UNSPECIFIED.);
#799=B_SPLINE_CURVE_WITH_KNOTS('',3,(#18653,#18654,#18655,#18656),
 .UNSPECIFIED.,.F.,.F.,(4,4),(9.85750350611301,10.4271318523291),
 .UNSPECIFIED.);
#800=B_SPLINE_CURVE_WITH_KNOTS('',3,(#18660,#18661,#18662,#18663),
 .UNSPECIFIED.,.F.,.F.,(4,4),(0.27539863731415,0.845026983530265),
 .UNSPECIFIED.);
#801=B_SPLINE_CURVE_WITH_KNOTS('',3,(#18681,#18682,#18683,#18684),
 .UNSPECIFIED.,.F.,.F.,(4,4),(-0.851674123393175,-0.27539863731415),
 .UNSPECIFIED.);
#802=B_SPLINE_CURVE_WITH_KNOTS('',3,(#18685,#18686,#18687,#18688),
 .UNSPECIFIED.,.F.,.F.,(4,4),(-0.618489359031386,-0.0112334529114389),
 .UNSPECIFIED.);
#803=B_SPLINE_CURVE_WITH_KNOTS('',3,(#18768,#18769,#18770,#18771),
 .UNSPECIFIED.,.F.,.F.,(4,4),(0.0112755522169305,0.618164468641375),
 .UNSPECIFIED.);
#804=B_SPLINE_CURVE_WITH_KNOTS('',3,(#18792,#18793,#18794,#18795),
 .UNSPECIFIED.,.F.,.F.,(4,4),(-0.618164468641375,-0.0112755522169305),
 .UNSPECIFIED.);
#805=B_SPLINE_CURVE_WITH_KNOTS('',3,(#18881,#18882,#18883,#18884),
 .UNSPECIFIED.,.F.,.F.,(4,4),(5.55111512312578E-17,0.618489359031386),
 .UNSPECIFIED.);
#806=B_SPLINE_CURVE_WITH_KNOTS('',3,(#18885,#18886,#18887,#18888),
 .UNSPECIFIED.,.F.,.F.,(4,4),(-0.618489359031386,-0.00110654915602034),
 .UNSPECIFIED.);
#807=B_SPLINE_CURVE_WITH_KNOTS('',3,(#18924,#18925,#18926,#18927,#18928),
 .UNSPECIFIED.,.F.,.F.,(4,1,4),(-10.4271318523291,-4.63063308449434,-0.283259008618247),
 .UNSPECIFIED.);
#808=B_SPLINE_CURVE_WITH_KNOTS('',3,(#18929,#18930,#18931,#18932,#18933),
 .UNSPECIFIED.,.F.,.F.,(4,1,4),(0.283259011433087,4.63063308449434,10.4271318523291),
 .UNSPECIFIED.);
#809=B_SPLINE_CURVE_WITH_KNOTS('',3,(#18954,#18955,#18956,#18957),
 .UNSPECIFIED.,.F.,.F.,(4,4),(0.000779732613545348,0.618164468641375),
 .UNSPECIFIED.);
#810=B_SPLINE_CURVE_WITH_KNOTS('',3,(#18958,#18959,#18960,#18961),
 .UNSPECIFIED.,.F.,.F.,(4,4),(-0.618164468641375,-4.9439619065339E-17),
 .UNSPECIFIED.);
#811=B_SPLINE_CURVE_WITH_KNOTS('',3,(#18982,#18983,#18984,#18985),
 .UNSPECIFIED.,.F.,.F.,(4,4),(3.0964814046186E-16,0.618164468641375),
 .UNSPECIFIED.);
#812=B_SPLINE_CURVE_WITH_KNOTS('',3,(#18986,#18987,#18988,#18989),
 .UNSPECIFIED.,.F.,.F.,(4,4),(-0.618164468641375,-0.0007797326135453),
 .UNSPECIFIED.);
#813=B_SPLINE_CURVE_WITH_KNOTS('',3,(#19015,#19016,#19017,#19018,#19019),
 .UNSPECIFIED.,.F.,.F.,(4,1,4),(-10.419271481025,-4.62277271319024,-0.27539863731415),
 .UNSPECIFIED.);
#814=B_SPLINE_CURVE_WITH_KNOTS('',3,(#19020,#19021,#19022,#19023,#19024),
 .UNSPECIFIED.,.F.,.F.,(4,1,4),(0.27539863731415,4.62277271319024,10.419271481025),
 .UNSPECIFIED.);
#815=B_SPLINE_CURVE_WITH_KNOTS('',3,(#19045,#19046,#19047,#19048),
 .UNSPECIFIED.,.F.,.F.,(4,4),(0.00110654915602046,0.618489359031386),
 .UNSPECIFIED.);
#816=B_SPLINE_CURVE_WITH_KNOTS('',3,(#19049,#19050,#19051,#19052),
 .UNSPECIFIED.,.F.,.F.,(4,4),(-0.618489359031386,6.93889390390723E-18),
 .UNSPECIFIED.);
#1231=PLANE('',#10380);
#1232=PLANE('',#10384);
#1233=PLANE('',#10385);
#1234=PLANE('',#10386);
#1235=PLANE('',#10387);
#1236=PLANE('',#10388);
#1237=PLANE('',#10389);
#1238=PLANE('',#10390);
#1239=PLANE('',#10392);
#1240=PLANE('',#10393);
#1241=PLANE('',#10394);
#1242=PLANE('',#10395);
#1243=PLANE('',#10396);
#1244=PLANE('',#10397);
#1245=PLANE('',#10398);
#1246=PLANE('',#10414);
#1247=PLANE('',#10415);
#1248=PLANE('',#10416);
#1249=PLANE('',#10417);
#1250=PLANE('',#10418);
#1251=PLANE('',#10419);
#1252=PLANE('',#10420);
#1253=PLANE('',#10421);
#1254=PLANE('',#10423);
#1255=PLANE('',#10425);
#1256=PLANE('',#10426);
#1257=PLANE('',#10427);
#1258=PLANE('',#10428);
#1259=PLANE('',#10429);
#1260=PLANE('',#10430);
#1261=PLANE('',#10431);
#1262=PLANE('',#10432);
#1263=PLANE('',#10433);
#1264=PLANE('',#10434);
#1265=PLANE('',#10435);
#1266=PLANE('',#10439);
#1267=PLANE('',#10441);
#1268=PLANE('',#10442);
#1269=PLANE('',#10443);
#1270=PLANE('',#10444);
#1271=PLANE('',#10445);
#1272=PLANE('',#10446);
#1273=PLANE('',#10448);
#1274=PLANE('',#10465);
#1275=PLANE('',#10484);
#1276=PLANE('',#10485);
#1277=PLANE('',#10486);
#1622=FACE_OUTER_BOUND('',#2207,.T.);
#1623=FACE_OUTER_BOUND('',#2208,.T.);
#1624=FACE_OUTER_BOUND('',#2209,.T.);
#1625=FACE_OUTER_BOUND('',#2210,.T.);
#1626=FACE_OUTER_BOUND('',#2211,.T.);
#1627=FACE_OUTER_BOUND('',#2212,.T.);
#1628=FACE_OUTER_BOUND('',#2213,.T.);
#1629=FACE_OUTER_BOUND('',#2217,.T.);
#1630=FACE_OUTER_BOUND('',#2218,.T.);
#1631=FACE_OUTER_BOUND('',#2219,.T.);
#1632=FACE_OUTER_BOUND('',#2220,.T.);
#1633=FACE_OUTER_BOUND('',#2221,.T.);
#1634=FACE_OUTER_BOUND('',#2222,.T.);
#1635=FACE_OUTER_BOUND('',#2223,.T.);
#1636=FACE_OUTER_BOUND('',#2225,.T.);
#1637=FACE_OUTER_BOUND('',#2226,.T.);
#1638=FACE_OUTER_BOUND('',#2227,.T.);
#1639=FACE_OUTER_BOUND('',#2228,.T.);
#1640=FACE_OUTER_BOUND('',#2229,.T.);
#1641=FACE_OUTER_BOUND('',#2230,.T.);
#1642=FACE_OUTER_BOUND('',#2231,.T.);
#1643=FACE_OUTER_BOUND('',#2233,.T.);
#1644=FACE_OUTER_BOUND('',#2234,.T.);
#1645=FACE_OUTER_BOUND('',#2235,.T.);
#1646=FACE_OUTER_BOUND('',#2236,.T.);
#1647=FACE_OUTER_BOUND('',#2237,.T.);
#1648=FACE_OUTER_BOUND('',#2238,.T.);
#1649=FACE_OUTER_BOUND('',#2239,.T.);
#1650=FACE_OUTER_BOUND('',#2240,.T.);
#1651=FACE_OUTER_BOUND('',#2241,.T.);
#1652=FACE_OUTER_BOUND('',#2242,.T.);
#1653=FACE_OUTER_BOUND('',#2243,.T.);
#1654=FACE_OUTER_BOUND('',#2244,.T.);
#1655=FACE_OUTER_BOUND('',#2245,.T.);
#1656=FACE_OUTER_BOUND('',#2246,.T.);
#1657=FACE_OUTER_BOUND('',#2248,.T.);
#1658=FACE_OUTER_BOUND('',#2250,.T.);
#1659=FACE_OUTER_BOUND('',#2251,.T.);
#1660=FACE_OUTER_BOUND('',#2252,.T.);
#1661=FACE_OUTER_BOUND('',#2253,.T.);
#1662=FACE_OUTER_BOUND('',#2254,.T.);
#1663=FACE_OUTER_BOUND('',#2255,.T.);
#1664=FACE_OUTER_BOUND('',#2256,.T.);
#1665=FACE_OUTER_BOUND('',#2257,.T.);
#1666=FACE_OUTER_BOUND('',#2258,.T.);
#1667=FACE_OUTER_BOUND('',#2259,.T.);
#1668=FACE_OUTER_BOUND('',#2260,.T.);
#1669=FACE_OUTER_BOUND('',#2262,.T.);
#1670=FACE_OUTER_BOUND('',#2263,.T.);
#1671=FACE_OUTER_BOUND('',#2264,.T.);
#1672=FACE_OUTER_BOUND('',#2265,.T.);
#1673=FACE_OUTER_BOUND('',#2266,.T.);
#1674=FACE_OUTER_BOUND('',#2267,.T.);
#1675=FACE_OUTER_BOUND('',#2268,.T.);
#1676=FACE_OUTER_BOUND('',#2269,.T.);
#1677=FACE_OUTER_BOUND('',#2270,.T.);
#1678=FACE_OUTER_BOUND('',#2271,.T.);
#1679=FACE_OUTER_BOUND('',#2272,.T.);
#1680=FACE_OUTER_BOUND('',#2273,.T.);
#1681=FACE_OUTER_BOUND('',#2274,.T.);
#1682=FACE_OUTER_BOUND('',#2275,.T.);
#1683=FACE_OUTER_BOUND('',#2276,.T.);
#1684=FACE_OUTER_BOUND('',#2277,.T.);
#1685=FACE_OUTER_BOUND('',#2278,.T.);
#1686=FACE_OUTER_BOUND('',#2279,.T.);
#1687=FACE_OUTER_BOUND('',#2280,.T.);
#1688=FACE_OUTER_BOUND('',#2281,.T.);
#1689=FACE_OUTER_BOUND('',#2285,.T.);
#1690=FACE_OUTER_BOUND('',#2286,.T.);
#1691=FACE_OUTER_BOUND('',#2287,.T.);
#1692=FACE_OUTER_BOUND('',#2288,.T.);
#1693=FACE_OUTER_BOUND('',#2289,.T.);
#1694=FACE_OUTER_BOUND('',#2290,.T.);
#1695=FACE_OUTER_BOUND('',#2291,.T.);
#1696=FACE_OUTER_BOUND('',#2292,.T.);
#1697=FACE_OUTER_BOUND('',#2293,.T.);
#1698=FACE_OUTER_BOUND('',#2294,.T.);
#1699=FACE_OUTER_BOUND('',#2295,.T.);
#1700=FACE_OUTER_BOUND('',#2296,.T.);
#1701=FACE_OUTER_BOUND('',#2297,.T.);
#1702=FACE_OUTER_BOUND('',#2298,.T.);
#1703=FACE_OUTER_BOUND('',#2299,.T.);
#1704=FACE_OUTER_BOUND('',#2300,.T.);
#1705=FACE_OUTER_BOUND('',#2301,.T.);
#1706=FACE_OUTER_BOUND('',#2302,.T.);
#1707=FACE_OUTER_BOUND('',#2303,.T.);
#1708=FACE_OUTER_BOUND('',#2304,.T.);
#1709=FACE_OUTER_BOUND('',#2305,.T.);
#1710=FACE_OUTER_BOUND('',#2306,.T.);
#1711=FACE_OUTER_BOUND('',#2307,.T.);
#1712=FACE_OUTER_BOUND('',#2308,.T.);
#1713=FACE_OUTER_BOUND('',#2309,.T.);
#1714=FACE_OUTER_BOUND('',#2310,.T.);
#1715=FACE_OUTER_BOUND('',#2311,.T.);
#1716=FACE_OUTER_BOUND('',#2312,.T.);
#1717=FACE_OUTER_BOUND('',#2313,.T.);
#1718=FACE_OUTER_BOUND('',#2314,.T.);
#1719=FACE_OUTER_BOUND('',#2315,.T.);
#1720=FACE_OUTER_BOUND('',#2316,.T.);
#1721=FACE_OUTER_BOUND('',#2317,.T.);
#1722=FACE_OUTER_BOUND('',#2318,.T.);
#1723=FACE_OUTER_BOUND('',#2325,.T.);
#1724=FACE_OUTER_BOUND('',#2326,.T.);
#2207=EDGE_LOOP('',(#7965,#7966));
#2208=EDGE_LOOP('',(#7967,#7968));
#2209=EDGE_LOOP('',(#7969,#7970));
#2210=EDGE_LOOP('',(#7971,#7972));
#2211=EDGE_LOOP('',(#7973,#7974,#7975,#7976,#7977,#7978));
#2212=EDGE_LOOP('',(#7979,#7980,#7981,#7982,#7983,#7984));
#2213=EDGE_LOOP('',(#7985,#7986,#7987,#7988,#7989,#7990,#7991,#7992));
#2214=EDGE_LOOP('',(#7993));
#2215=EDGE_LOOP('',(#7994));
#2216=EDGE_LOOP('',(#7995));
#2217=EDGE_LOOP('',(#7996,#7997,#7998,#7999));
#2218=EDGE_LOOP('',(#8000,#8001,#8002,#8003));
#2219=EDGE_LOOP('',(#8004,#8005,#8006,#8007));
#2220=EDGE_LOOP('',(#8008,#8009,#8010,#8011));
#2221=EDGE_LOOP('',(#8012,#8013,#8014,#8015));
#2222=EDGE_LOOP('',(#8016,#8017,#8018,#8019));
#2223=EDGE_LOOP('',(#8020,#8021,#8022,#8023,#8024,#8025));
#2224=EDGE_LOOP('',(#8026));
#2225=EDGE_LOOP('',(#8027,#8028,#8029,#8030));
#2226=EDGE_LOOP('',(#8031,#8032,#8033,#8034));
#2227=EDGE_LOOP('',(#8035,#8036,#8037,#8038));
#2228=EDGE_LOOP('',(#8039,#8040,#8041,#8042));
#2229=EDGE_LOOP('',(#8043,#8044,#8045,#8046));
#2230=EDGE_LOOP('',(#8047,#8048,#8049,#8050));
#2231=EDGE_LOOP('',(#8051,#8052,#8053,#8054,#8055,#8056));
#2232=EDGE_LOOP('',(#8057));
#2233=EDGE_LOOP('',(#8058,#8059,#8060,#8061));
#2234=EDGE_LOOP('',(#8062,#8063,#8064,#8065));
#2235=EDGE_LOOP('',(#8066,#8067,#8068,#8069));
#2236=EDGE_LOOP('',(#8070,#8071,#8072,#8073));
#2237=EDGE_LOOP('',(#8074,#8075,#8076,#8077));
#2238=EDGE_LOOP('',(#8078,#8079,#8080,#8081));
#2239=EDGE_LOOP('',(#8082,#8083,#8084,#8085));
#2240=EDGE_LOOP('',(#8086,#8087,#8088,#8089));
#2241=EDGE_LOOP('',(#8090,#8091,#8092,#8093));
#2242=EDGE_LOOP('',(#8094,#8095,#8096,#8097));
#2243=EDGE_LOOP('',(#8098,#8099,#8100,#8101));
#2244=EDGE_LOOP('',(#8102,#8103,#8104,#8105));
#2245=EDGE_LOOP('',(#8106,#8107,#8108,#8109));
#2246=EDGE_LOOP('',(#8110));
#2247=EDGE_LOOP('',(#8111));
#2248=EDGE_LOOP('',(#8112));
#2249=EDGE_LOOP('',(#8113));
#2250=EDGE_LOOP('',(#8114,#8115,#8116,#8117));
#2251=EDGE_LOOP('',(#8118,#8119,#8120,#8121));
#2252=EDGE_LOOP('',(#8122,#8123,#8124,#8125));
#2253=EDGE_LOOP('',(#8126,#8127,#8128,#8129));
#2254=EDGE_LOOP('',(#8130,#8131,#8132,#8133));
#2255=EDGE_LOOP('',(#8134,#8135,#8136,#8137,#8138,#8139));
#2256=EDGE_LOOP('',(#8140,#8141,#8142,#8143,#8144,#8145,#8146,#8147,#8148,
#8149));
#2257=EDGE_LOOP('',(#8150,#8151,#8152,#8153,#8154,#8155,#8156,#8157,#8158,
#8159));
#2258=EDGE_LOOP('',(#8160,#8161,#8162,#8163,#8164,#8165,#8166,#8167,#8168,
#8169));
#2259=EDGE_LOOP('',(#8170,#8171,#8172,#8173,#8174,#8175,#8176,#8177));
#2260=EDGE_LOOP('',(#8178,#8179,#8180,#8181,#8182,#8183,#8184,#8185,#8186,
#8187,#8188,#8189,#8190,#8191,#8192,#8193,#8194,#8195,#8196,#8197,#8198,
#8199,#8200,#8201,#8202,#8203,#8204,#8205,#8206,#8207,#8208,#8209,#8210,
#8211,#8212,#8213,#8214,#8215,#8216,#8217,#8218,#8219));
#2261=EDGE_LOOP('',(#8220,#8221,#8222,#8223,#8224,#8225));
#2262=EDGE_LOOP('',(#8226,#8227,#8228,#8229));
#2263=EDGE_LOOP('',(#8230,#8231,#8232,#8233));
#2264=EDGE_LOOP('',(#8234,#8235,#8236,#8237,#8238,#8239));
#2265=EDGE_LOOP('',(#8240,#8241,#8242,#8243));
#2266=EDGE_LOOP('',(#8244,#8245,#8246,#8247));
#2267=EDGE_LOOP('',(#8248,#8249,#8250,#8251,#8252,#8253));
#2268=EDGE_LOOP('',(#8254,#8255,#8256,#8257));
#2269=EDGE_LOOP('',(#8258,#8259,#8260,#8261));
#2270=EDGE_LOOP('',(#8262,#8263,#8264,#8265));
#2271=EDGE_LOOP('',(#8266,#8267,#8268,#8269));
#2272=EDGE_LOOP('',(#8270,#8271,#8272,#8273,#8274,#8275,#8276,#8277,#8278,
#8279));
#2273=EDGE_LOOP('',(#8280,#8281,#8282,#8283));
#2274=EDGE_LOOP('',(#8284,#8285,#8286,#8287));
#2275=EDGE_LOOP('',(#8288,#8289,#8290,#8291));
#2276=EDGE_LOOP('',(#8292,#8293,#8294,#8295));
#2277=EDGE_LOOP('',(#8296,#8297,#8298,#8299));
#2278=EDGE_LOOP('',(#8300,#8301,#8302,#8303,#8304,#8305,#8306,#8307,#8308,
#8309));
#2279=EDGE_LOOP('',(#8310,#8311,#8312,#8313));
#2280=EDGE_LOOP('',(#8314,#8315,#8316,#8317,#8318,#8319));
#2281=EDGE_LOOP('',(#8320,#8321,#8322,#8323,#8324,#8325,#8326,#8327));
#2282=EDGE_LOOP('',(#8328));
#2283=EDGE_LOOP('',(#8329));
#2284=EDGE_LOOP('',(#8330));
#2285=EDGE_LOOP('',(#8331,#8332,#8333,#8334));
#2286=EDGE_LOOP('',(#8335,#8336,#8337,#8338,#8339,#8340,#8341,#8342,#8343,
#8344));
#2287=EDGE_LOOP('',(#8345,#8346,#8347,#8348));
#2288=EDGE_LOOP('',(#8349,#8350,#8351,#8352));
#2289=EDGE_LOOP('',(#8353,#8354,#8355,#8356));
#2290=EDGE_LOOP('',(#8357,#8358,#8359,#8360));
#2291=EDGE_LOOP('',(#8361,#8362,#8363,#8364));
#2292=EDGE_LOOP('',(#8365,#8366,#8367));
#2293=EDGE_LOOP('',(#8368,#8369,#8370));
#2294=EDGE_LOOP('',(#8371,#8372,#8373));
#2295=EDGE_LOOP('',(#8374,#8375,#8376,#8377));
#2296=EDGE_LOOP('',(#8378,#8379,#8380,#8381));
#2297=EDGE_LOOP('',(#8382,#8383,#8384));
#2298=EDGE_LOOP('',(#8385,#8386,#8387,#8388));
#2299=EDGE_LOOP('',(#8389,#8390,#8391,#8392));
#2300=EDGE_LOOP('',(#8393,#8394,#8395,#8396));
#2301=EDGE_LOOP('',(#8397,#8398,#8399,#8400));
#2302=EDGE_LOOP('',(#8401,#8402,#8403,#8404));
#2303=EDGE_LOOP('',(#8405,#8406,#8407,#8408));
#2304=EDGE_LOOP('',(#8409,#8410,#8411));
#2305=EDGE_LOOP('',(#8412,#8413,#8414));
#2306=EDGE_LOOP('',(#8415,#8416,#8417));
#2307=EDGE_LOOP('',(#8418,#8419,#8420,#8421));
#2308=EDGE_LOOP('',(#8422,#8423,#8424,#8425));
#2309=EDGE_LOOP('',(#8426,#8427,#8428));
#2310=EDGE_LOOP('',(#8429,#8430,#8431,#8432));
#2311=EDGE_LOOP('',(#8433,#8434,#8435,#8436));
#2312=EDGE_LOOP('',(#8437,#8438,#8439,#8440));
#2313=EDGE_LOOP('',(#8441,#8442,#8443,#8444));
#2314=EDGE_LOOP('',(#8445,#8446,#8447,#8448));
#2315=EDGE_LOOP('',(#8449,#8450,#8451,#8452));
#2316=EDGE_LOOP('',(#8453,#8454,#8455,#8456));
#2317=EDGE_LOOP('',(#8457,#8458,#8459,#8460,#8461,#8462,#8463,#8464));
#2318=EDGE_LOOP('',(#8465,#8466,#8467,#8468));
#2319=EDGE_LOOP('',(#8469,#8470,#8471,#8472,#8473,#8474));
#2320=EDGE_LOOP('',(#8475,#8476,#8477,#8478,#8479,#8480));
#2321=EDGE_LOOP('',(#8481));
#2322=EDGE_LOOP('',(#8482));
#2323=EDGE_LOOP('',(#8483));
#2324=EDGE_LOOP('',(#8484));
#2325=EDGE_LOOP('',(#8485,#8486,#8487,#8488));
#2326=EDGE_LOOP('',(#8489,#8490,#8491,#8492));
#2825=LINE('',#17278,#3413);
#2826=LINE('',#17280,#3414);
#2827=LINE('',#17294,#3415);
#2828=LINE('',#17296,#3416);
#2829=LINE('',#17298,#3417);
#2830=LINE('',#17299,#3418);
#2831=LINE('',#17302,#3419);
#2832=LINE('',#17304,#3420);
#2833=LINE('',#17305,#3421);
#2834=LINE('',#17308,#3422);
#2835=LINE('',#17310,#3423);
#2836=LINE('',#17311,#3424);
#2837=LINE('',#17314,#3425);
#2838=LINE('',#17316,#3426);
#2839=LINE('',#17317,#3427);
#2840=LINE('',#17320,#3428);
#2841=LINE('',#17322,#3429);
#2842=LINE('',#17323,#3430);
#2843=LINE('',#17325,#3431);
#2844=LINE('',#17326,#3432);
#2845=LINE('',#17333,#3433);
#2846=LINE('',#17335,#3434);
#2847=LINE('',#17337,#3435);
#2848=LINE('',#17338,#3436);
#2849=LINE('',#17341,#3437);
#2850=LINE('',#17343,#3438);
#2851=LINE('',#17344,#3439);
#2852=LINE('',#17347,#3440);
#2853=LINE('',#17349,#3441);
#2854=LINE('',#17350,#3442);
#2855=LINE('',#17353,#3443);
#2856=LINE('',#17355,#3444);
#2857=LINE('',#17356,#3445);
#2858=LINE('',#17359,#3446);
#2859=LINE('',#17361,#3447);
#2860=LINE('',#17362,#3448);
#2861=LINE('',#17364,#3449);
#2862=LINE('',#17365,#3450);
#2863=LINE('',#17372,#3451);
#2864=LINE('',#17377,#3452);
#2865=LINE('',#17383,#3453);
#2866=LINE('',#17388,#3454);
#2867=LINE('',#17391,#3455);
#2868=LINE('',#17395,#3456);
#2869=LINE('',#17400,#3457);
#2870=LINE('',#17402,#3458);
#2871=LINE('',#17404,#3459);
#2872=LINE('',#17405,#3460);
#2873=LINE('',#17409,#3461);
#2874=LINE('',#17411,#3462);
#2875=LINE('',#17413,#3463);
#2876=LINE('',#17414,#3464);
#2877=LINE('',#17418,#3465);
#2878=LINE('',#17420,#3466);
#2879=LINE('',#17422,#3467);
#2880=LINE('',#17423,#3468);
#2881=LINE('',#17427,#3469);
#2882=LINE('',#17429,#3470);
#2883=LINE('',#17431,#3471);
#2884=LINE('',#17432,#3472);
#2885=LINE('',#17436,#3473);
#2886=LINE('',#17438,#3474);
#2887=LINE('',#17440,#3475);
#2888=LINE('',#17441,#3476);
#2889=LINE('',#17445,#3477);
#2890=LINE('',#17447,#3478);
#2891=LINE('',#17449,#3479);
#2892=LINE('',#17450,#3480);
#2893=LINE('',#17454,#3481);
#2894=LINE('',#17456,#3482);
#2895=LINE('',#17458,#3483);
#2896=LINE('',#17459,#3484);
#2897=LINE('',#17467,#3485);
#2898=LINE('',#17468,#3486);
#2899=LINE('',#17470,#3487);
#2900=LINE('',#17471,#3488);
#2901=LINE('',#17473,#3489);
#2902=LINE('',#17474,#3490);
#2903=LINE('',#17477,#3491);
#2904=LINE('',#17479,#3492);
#2905=LINE('',#17480,#3493);
#2906=LINE('',#17483,#3494);
#2907=LINE('',#17485,#3495);
#2908=LINE('',#17486,#3496);
#2909=LINE('',#17490,#3497);
#2910=LINE('',#17534,#3498);
#2911=LINE('',#17577,#3499);
#2912=LINE('',#17580,#3500);
#2913=LINE('',#17618,#3501);
#2914=LINE('',#17655,#3502);
#2915=LINE('',#17658,#3503);
#2916=LINE('',#17666,#3504);
#2917=LINE('',#17703,#3505);
#2918=LINE('',#17706,#3506);
#2919=LINE('',#17713,#3507);
#2920=LINE('',#17719,#3508);
#2921=LINE('',#17730,#3509);
#2922=LINE('',#17739,#3510);
#2923=LINE('',#17745,#3511);
#2924=LINE('',#17780,#3512);
#2925=LINE('',#17851,#3513);
#2926=LINE('',#17921,#3514);
#2927=LINE('',#17953,#3515);
#2928=LINE('',#17959,#3516);
#2929=LINE('',#17968,#3517);
#2930=LINE('',#18005,#3518);
#2931=LINE('',#18040,#3519);
#2932=LINE('',#18042,#3520);
#2933=LINE('',#18046,#3521);
#2934=LINE('',#18092,#3522);
#2935=LINE('',#18218,#3523);
#2936=LINE('',#18298,#3524);
#2937=LINE('',#18460,#3525);
#2938=LINE('',#18570,#3526);
#2939=LINE('',#18659,#3527);
#2940=LINE('',#18747,#3528);
#2941=LINE('',#18859,#3529);
#2942=LINE('',#18860,#3530);
#2943=LINE('',#18897,#3531);
#2944=LINE('',#18898,#3532);
#3413=VECTOR('',#11757,1.);
#3414=VECTOR('',#11758,1.);
#3415=VECTOR('',#11767,1.);
#3416=VECTOR('',#11768,1.);
#3417=VECTOR('',#11769,1.);
#3418=VECTOR('',#11770,1.);
#3419=VECTOR('',#11773,1.);
#3420=VECTOR('',#11774,1.);
#3421=VECTOR('',#11775,1.);
#3422=VECTOR('',#11778,1.);
#3423=VECTOR('',#11779,1.);
#3424=VECTOR('',#11780,1.);
#3425=VECTOR('',#11783,1.);
#3426=VECTOR('',#11784,1.);
#3427=VECTOR('',#11785,1.);
#3428=VECTOR('',#11788,1.);
#3429=VECTOR('',#11789,1.);
#3430=VECTOR('',#11790,1.);
#3431=VECTOR('',#11793,1.);
#3432=VECTOR('',#11794,1.);
#3433=VECTOR('',#11801,1.);
#3434=VECTOR('',#11802,1.);
#3435=VECTOR('',#11803,1.);
#3436=VECTOR('',#11804,1.);
#3437=VECTOR('',#11807,1.);
#3438=VECTOR('',#11808,1.);
#3439=VECTOR('',#11809,1.);
#3440=VECTOR('',#11812,1.);
#3441=VECTOR('',#11813,1.);
#3442=VECTOR('',#11814,1.);
#3443=VECTOR('',#11817,1.);
#3444=VECTOR('',#11818,1.);
#3445=VECTOR('',#11819,1.);
#3446=VECTOR('',#11822,1.);
#3447=VECTOR('',#11823,1.);
#3448=VECTOR('',#11824,1.);
#3449=VECTOR('',#11827,1.);
#3450=VECTOR('',#11828,1.);
#3451=VECTOR('',#11837,0.15);
#3452=VECTOR('',#11842,0.15);
#3453=VECTOR('',#11849,0.15);
#3454=VECTOR('',#11856,0.15);
#3455=VECTOR('',#11859,0.17);
#3456=VECTOR('',#11864,0.17);
#3457=VECTOR('',#11869,1.);
#3458=VECTOR('',#11870,1.);
#3459=VECTOR('',#11871,1.);
#3460=VECTOR('',#11872,1.);
#3461=VECTOR('',#11875,1.);
#3462=VECTOR('',#11876,1.);
#3463=VECTOR('',#11877,1.);
#3464=VECTOR('',#11878,1.);
#3465=VECTOR('',#11881,1.);
#3466=VECTOR('',#11882,1.);
#3467=VECTOR('',#11883,1.);
#3468=VECTOR('',#11884,1.);
#3469=VECTOR('',#11887,1.);
#3470=VECTOR('',#11888,1.);
#3471=VECTOR('',#11889,1.);
#3472=VECTOR('',#11890,1.);
#3473=VECTOR('',#11893,1.);
#3474=VECTOR('',#11894,1.);
#3475=VECTOR('',#11895,1.);
#3476=VECTOR('',#11896,1.);
#3477=VECTOR('',#11899,1.);
#3478=VECTOR('',#11900,1.);
#3479=VECTOR('',#11901,1.);
#3480=VECTOR('',#11902,1.);
#3481=VECTOR('',#11905,1.);
#3482=VECTOR('',#11906,1.);
#3483=VECTOR('',#11907,1.);
#3484=VECTOR('',#11908,1.);
#3485=VECTOR('',#11919,1.);
#3486=VECTOR('',#11920,1.);
#3487=VECTOR('',#11923,1.);
#3488=VECTOR('',#11924,1.);
#3489=VECTOR('',#11927,1.);
#3490=VECTOR('',#11928,1.);
#3491=VECTOR('',#11931,1.);
#3492=VECTOR('',#11932,1.);
#3493=VECTOR('',#11933,1.);
#3494=VECTOR('',#11936,1.);
#3495=VECTOR('',#11937,1.);
#3496=VECTOR('',#11938,1.);
#3497=VECTOR('',#11941,1.);
#3498=VECTOR('',#11944,1.);
#3499=VECTOR('',#11945,1.);
#3500=VECTOR('',#11948,1.);
#3501=VECTOR('',#11949,1.);
#3502=VECTOR('',#11950,1.);
#3503=VECTOR('',#11953,1.);
#3504=VECTOR('',#11954,1.);
#3505=VECTOR('',#11955,1.);
#3506=VECTOR('',#11958,1.);
#3507=VECTOR('',#11959,1.);
#3508=VECTOR('',#11960,1.);
#3509=VECTOR('',#11963,1.);
#3510=VECTOR('',#11964,1.);
#3511=VECTOR('',#11965,1.);
#3512=VECTOR('',#11966,1.);
#3513=VECTOR('',#11967,1.);
#3514=VECTOR('',#11968,1.);
#3515=VECTOR('',#11969,1.);
#3516=VECTOR('',#11970,1.);
#3517=VECTOR('',#11971,1.);
#3518=VECTOR('',#11972,1.);
#3519=VECTOR('',#11973,1.);
#3520=VECTOR('',#11976,0.4);
#3521=VECTOR('',#11981,0.4);
#3522=VECTOR('',#11984,1.);
#3523=VECTOR('',#11989,1.);
#3524=VECTOR('',#11992,1.);
#3525=VECTOR('',#11997,1.);
#3526=VECTOR('',#12002,1.);
#3527=VECTOR('',#12007,1.);
#3528=VECTOR('',#12040,1.);
#3529=VECTOR('',#12069,1.);
#3530=VECTOR('',#12070,1.);
#3531=VECTOR('',#12081,1.);
#3532=VECTOR('',#12082,1.);
#3739=CIRCLE('',#10373,0.25);
#3740=CIRCLE('',#10375,0.25);
#3741=CIRCLE('',#10377,0.25);
#3742=CIRCLE('',#10379,0.25);
#3743=CIRCLE('',#10381,0.15);
#3744=CIRCLE('',#10382,0.15);
#3745=CIRCLE('',#10383,0.4);
#3746=CIRCLE('',#10391,0.17);
#3747=CIRCLE('',#10399,0.17);
#3748=CIRCLE('',#10401,0.15);
#3749=CIRCLE('',#10403,0.15);
#3750=CIRCLE('',#10404,0.15);
#3751=CIRCLE('',#10406,0.15);
#3752=CIRCLE('',#10407,0.15);
#3753=CIRCLE('',#10409,0.15);
#3754=CIRCLE('',#10411,0.17);
#3755=CIRCLE('',#10413,0.17);
#3756=CIRCLE('',#10422,0.4);
#3757=CIRCLE('',#10424,0.4);
#3758=CIRCLE('',#10438,0.4);
#3759=CIRCLE('',#10440,0.1);
#3760=CIRCLE('',#10447,0.0999999999999995);
#3761=CIRCLE('',#10449,0.1);
#3762=CIRCLE('',#10451,0.1);
#3763=CIRCLE('',#10452,0.1);
#3764=CIRCLE('',#10454,0.0999999999999999);
#3765=CIRCLE('',#10455,0.0999999999999998);
#3766=CIRCLE('',#10456,0.0999999999999998);
#3767=CIRCLE('',#10458,0.0999999999999994);
#3768=CIRCLE('',#10459,0.0999999999999993);
#3769=CIRCLE('',#10462,0.0999999999999999);
#3770=CIRCLE('',#10463,0.1);
#3771=CIRCLE('',#10467,0.3);
#3772=CIRCLE('',#10468,0.3);
#3773=CIRCLE('',#10469,0.3);
#3774=CIRCLE('',#10471,0.3);
#3775=CIRCLE('',#10472,0.3);
#3776=CIRCLE('',#10473,0.3);
#3777=CIRCLE('',#10475,0.3);
#3778=CIRCLE('',#10476,0.299999999999999);
#3779=CIRCLE('',#10477,0.3);
#3780=CIRCLE('',#10480,0.3);
#3781=CIRCLE('',#10481,0.3);
#3782=CIRCLE('',#10482,0.3);
#4387=VERTEX_POINT('',#16985);
#4388=VERTEX_POINT('',#16986);
#4389=VERTEX_POINT('',#17013);
#4390=VERTEX_POINT('',#17014);
#4391=VERTEX_POINT('',#17037);
#4392=VERTEX_POINT('',#17038);
#4393=VERTEX_POINT('',#17061);
#4394=VERTEX_POINT('',#17062);
#4395=VERTEX_POINT('',#17108);
#4396=VERTEX_POINT('',#17113);
#4397=VERTEX_POINT('',#17142);
#4398=VERTEX_POINT('',#17147);
#4399=VERTEX_POINT('',#17200);
#4400=VERTEX_POINT('',#17205);
#4401=VERTEX_POINT('',#17234);
#4402=VERTEX_POINT('',#17239);
#4403=VERTEX_POINT('',#17273);
#4404=VERTEX_POINT('',#17279);
#4405=VERTEX_POINT('',#17285);
#4406=VERTEX_POINT('',#17287);
#4407=VERTEX_POINT('',#17289);
#4408=VERTEX_POINT('',#17292);
#4409=VERTEX_POINT('',#17293);
#4410=VERTEX_POINT('',#17295);
#4411=VERTEX_POINT('',#17297);
#4412=VERTEX_POINT('',#17301);
#4413=VERTEX_POINT('',#17303);
#4414=VERTEX_POINT('',#17307);
#4415=VERTEX_POINT('',#17309);
#4416=VERTEX_POINT('',#17313);
#4417=VERTEX_POINT('',#17315);
#4418=VERTEX_POINT('',#17319);
#4419=VERTEX_POINT('',#17321);
#4420=VERTEX_POINT('',#17328);
#4421=VERTEX_POINT('',#17331);
#4422=VERTEX_POINT('',#17332);
#4423=VERTEX_POINT('',#17334);
#4424=VERTEX_POINT('',#17336);
#4425=VERTEX_POINT('',#17340);
#4426=VERTEX_POINT('',#17342);
#4427=VERTEX_POINT('',#17346);
#4428=VERTEX_POINT('',#17348);
#4429=VERTEX_POINT('',#17352);
#4430=VERTEX_POINT('',#17354);
#4431=VERTEX_POINT('',#17358);
#4432=VERTEX_POINT('',#17360);
#4433=VERTEX_POINT('',#17367);
#4434=VERTEX_POINT('',#17370);
#4435=VERTEX_POINT('',#17374);
#4436=VERTEX_POINT('',#17376);
#4437=VERTEX_POINT('',#17380);
#4438=VERTEX_POINT('',#17382);
#4439=VERTEX_POINT('',#17386);
#4440=VERTEX_POINT('',#17390);
#4441=VERTEX_POINT('',#17394);
#4442=VERTEX_POINT('',#17398);
#4443=VERTEX_POINT('',#17399);
#4444=VERTEX_POINT('',#17401);
#4445=VERTEX_POINT('',#17403);
#4446=VERTEX_POINT('',#17407);
#4447=VERTEX_POINT('',#17408);
#4448=VERTEX_POINT('',#17410);
#4449=VERTEX_POINT('',#17412);
#4450=VERTEX_POINT('',#17416);
#4451=VERTEX_POINT('',#17417);
#4452=VERTEX_POINT('',#17419);
#4453=VERTEX_POINT('',#17421);
#4454=VERTEX_POINT('',#17425);
#4455=VERTEX_POINT('',#17426);
#4456=VERTEX_POINT('',#17428);
#4457=VERTEX_POINT('',#17430);
#4458=VERTEX_POINT('',#17434);
#4459=VERTEX_POINT('',#17435);
#4460=VERTEX_POINT('',#17437);
#4461=VERTEX_POINT('',#17439);
#4462=VERTEX_POINT('',#17443);
#4463=VERTEX_POINT('',#17444);
#4464=VERTEX_POINT('',#17446);
#4465=VERTEX_POINT('',#17448);
#4466=VERTEX_POINT('',#17452);
#4467=VERTEX_POINT('',#17453);
#4468=VERTEX_POINT('',#17455);
#4469=VERTEX_POINT('',#17457);
#4470=VERTEX_POINT('',#17461);
#4471=VERTEX_POINT('',#17464);
#4472=VERTEX_POINT('',#17476);
#4473=VERTEX_POINT('',#17478);
#4474=VERTEX_POINT('',#17482);
#4475=VERTEX_POINT('',#17484);
#4476=VERTEX_POINT('',#17488);
#4477=VERTEX_POINT('',#17489);
#4478=VERTEX_POINT('',#17491);
#4479=VERTEX_POINT('',#17533);
#4480=VERTEX_POINT('',#17541);
#4481=VERTEX_POINT('',#17570);
#4482=VERTEX_POINT('',#17579);
#4483=VERTEX_POINT('',#17581);
#4484=VERTEX_POINT('',#17588);
#4485=VERTEX_POINT('',#17617);
#4486=VERTEX_POINT('',#17619);
#4487=VERTEX_POINT('',#17648);
#4488=VERTEX_POINT('',#17657);
#4489=VERTEX_POINT('',#17665);
#4490=VERTEX_POINT('',#17667);
#4491=VERTEX_POINT('',#17696);
#4492=VERTEX_POINT('',#17705);
#4493=VERTEX_POINT('',#17707);
#4494=VERTEX_POINT('',#17712);
#4495=VERTEX_POINT('',#17714);
#4496=VERTEX_POINT('',#17729);
#4497=VERTEX_POINT('',#17738);
#4498=VERTEX_POINT('',#17744);
#4499=VERTEX_POINT('',#17746);
#4500=VERTEX_POINT('',#17779);
#4501=VERTEX_POINT('',#17781);
#4502=VERTEX_POINT('',#17813);
#4503=VERTEX_POINT('',#17818);
#4504=VERTEX_POINT('',#17850);
#4505=VERTEX_POINT('',#17852);
#4506=VERTEX_POINT('',#17884);
#4507=VERTEX_POINT('',#17889);
#4508=VERTEX_POINT('',#17922);
#4509=VERTEX_POINT('',#17948);
#4510=VERTEX_POINT('',#17954);
#4511=VERTEX_POINT('',#17960);
#4512=VERTEX_POINT('',#17969);
#4513=VERTEX_POINT('',#17970);
#4514=VERTEX_POINT('',#17975);
#4515=VERTEX_POINT('',#18004);
#4516=VERTEX_POINT('',#18006);
#4517=VERTEX_POINT('',#18035);
#4518=VERTEX_POINT('',#18044);
#4519=VERTEX_POINT('',#18048);
#4520=VERTEX_POINT('',#18055);
#4521=VERTEX_POINT('',#18062);
#4522=VERTEX_POINT('',#18091);
#4523=VERTEX_POINT('',#18157);
#4524=VERTEX_POINT('',#18206);
#4525=VERTEX_POINT('',#18213);
#4526=VERTEX_POINT('',#18251);
#4527=VERTEX_POINT('',#18261);
#4528=VERTEX_POINT('',#18268);
#4529=VERTEX_POINT('',#18297);
#4530=VERTEX_POINT('',#18299);
#4531=VERTEX_POINT('',#18424);
#4532=VERTEX_POINT('',#18431);
#4533=VERTEX_POINT('',#18533);
#4534=VERTEX_POINT('',#18540);
#4535=VERTEX_POINT('',#18569);
#4536=VERTEX_POINT('',#18571);
#4537=VERTEX_POINT('',#18622);
#4538=VERTEX_POINT('',#18651);
#4539=VERTEX_POINT('',#18658);
#4540=VERTEX_POINT('',#18680);
#4541=VERTEX_POINT('',#18715);
#4542=VERTEX_POINT('',#18743);
#4543=VERTEX_POINT('',#18838);
#4544=VERTEX_POINT('',#18839);
#4545=VERTEX_POINT('',#18841);
#4546=VERTEX_POINT('',#18845);
#4547=VERTEX_POINT('',#18846);
#4548=VERTEX_POINT('',#18848);
#4549=VERTEX_POINT('',#18852);
#4550=VERTEX_POINT('',#18853);
#4551=VERTEX_POINT('',#18855);
#4552=VERTEX_POINT('',#18890);
#4553=VERTEX_POINT('',#18891);
#4554=VERTEX_POINT('',#18893);
#5641=EDGE_CURVE('',#4387,#4388,#717,.T.);
#5642=EDGE_CURVE('',#4387,#4388,#3739,.T.);
#5643=EDGE_CURVE('',#4389,#4390,#718,.T.);
#5644=EDGE_CURVE('',#4389,#4390,#3740,.T.);
#5645=EDGE_CURVE('',#4391,#4392,#719,.T.);
#5646=EDGE_CURVE('',#4391,#4392,#3741,.T.);
#5647=EDGE_CURVE('',#4393,#4394,#720,.T.);
#5648=EDGE_CURVE('',#4393,#4394,#3742,.T.);
#5649=EDGE_CURVE('',#4395,#4390,#721,.T.);
#5650=EDGE_CURVE('',#4395,#4396,#722,.T.);
#5651=EDGE_CURVE('',#4397,#4396,#723,.T.);
#5652=EDGE_CURVE('',#4397,#4398,#724,.T.);
#5653=EDGE_CURVE('',#4389,#4398,#725,.T.);
#5654=EDGE_CURVE('',#4399,#4394,#726,.T.);
#5655=EDGE_CURVE('',#4399,#4400,#727,.T.);
#5656=EDGE_CURVE('',#4401,#4400,#728,.T.);
#5657=EDGE_CURVE('',#4401,#4402,#729,.T.);
#5658=EDGE_CURVE('',#4393,#4402,#730,.T.);
#5659=EDGE_CURVE('',#4387,#4403,#731,.T.);
#5660=EDGE_CURVE('',#4403,#4399,#2825,.T.);
#5661=EDGE_CURVE('',#4402,#4404,#2826,.T.);
#5662=EDGE_CURVE('',#4404,#4388,#732,.T.);
#5663=EDGE_CURVE('',#4405,#4405,#3743,.T.);
#5664=EDGE_CURVE('',#4406,#4406,#3744,.T.);
#5665=EDGE_CURVE('',#4407,#4407,#3745,.T.);
#5666=EDGE_CURVE('',#4408,#4409,#2827,.T.);
#5667=EDGE_CURVE('',#4408,#4410,#2828,.T.);
#5668=EDGE_CURVE('',#4410,#4411,#2829,.T.);
#5669=EDGE_CURVE('',#4409,#4411,#2830,.T.);
#5670=EDGE_CURVE('',#4412,#4408,#2831,.T.);
#5671=EDGE_CURVE('',#4412,#4413,#2832,.T.);
#5672=EDGE_CURVE('',#4413,#4410,#2833,.T.);
#5673=EDGE_CURVE('',#4414,#4412,#2834,.T.);
#5674=EDGE_CURVE('',#4414,#4415,#2835,.T.);
#5675=EDGE_CURVE('',#4415,#4413,#2836,.T.);
#5676=EDGE_CURVE('',#4416,#4414,#2837,.T.);
#5677=EDGE_CURVE('',#4416,#4417,#2838,.T.);
#5678=EDGE_CURVE('',#4417,#4415,#2839,.T.);
#5679=EDGE_CURVE('',#4418,#4416,#2840,.T.);
#5680=EDGE_CURVE('',#4418,#4419,#2841,.T.);
#5681=EDGE_CURVE('',#4419,#4417,#2842,.T.);
#5682=EDGE_CURVE('',#4409,#4418,#2843,.T.);
#5683=EDGE_CURVE('',#4411,#4419,#2844,.T.);
#5684=EDGE_CURVE('',#4420,#4420,#3746,.T.);
#5685=EDGE_CURVE('',#4421,#4422,#2845,.T.);
#5686=EDGE_CURVE('',#4421,#4423,#2846,.T.);
#5687=EDGE_CURVE('',#4423,#4424,#2847,.T.);
#5688=EDGE_CURVE('',#4422,#4424,#2848,.T.);
#5689=EDGE_CURVE('',#4425,#4421,#2849,.T.);
#5690=EDGE_CURVE('',#4425,#4426,#2850,.T.);
#5691=EDGE_CURVE('',#4426,#4423,#2851,.T.);
#5692=EDGE_CURVE('',#4427,#4425,#2852,.T.);
#5693=EDGE_CURVE('',#4427,#4428,#2853,.T.);
#5694=EDGE_CURVE('',#4428,#4426,#2854,.T.);
#5695=EDGE_CURVE('',#4429,#4427,#2855,.T.);
#5696=EDGE_CURVE('',#4429,#4430,#2856,.T.);
#5697=EDGE_CURVE('',#4430,#4428,#2857,.T.);
#5698=EDGE_CURVE('',#4431,#4429,#2858,.T.);
#5699=EDGE_CURVE('',#4431,#4432,#2859,.T.);
#5700=EDGE_CURVE('',#4432,#4430,#2860,.T.);
#5701=EDGE_CURVE('',#4422,#4431,#2861,.T.);
#5702=EDGE_CURVE('',#4424,#4432,#2862,.T.);
#5703=EDGE_CURVE('',#4433,#4433,#3747,.T.);
#5704=EDGE_CURVE('',#4434,#4434,#3748,.T.);
#5705=EDGE_CURVE('',#4434,#4405,#2863,.T.);
#5706=EDGE_CURVE('',#4435,#4435,#3749,.T.);
#5707=EDGE_CURVE('',#4435,#4436,#2864,.T.);
#5708=EDGE_CURVE('',#4436,#4436,#3750,.T.);
#5709=EDGE_CURVE('',#4437,#4437,#3751,.T.);
#5710=EDGE_CURVE('',#4437,#4438,#2865,.T.);
#5711=EDGE_CURVE('',#4438,#4438,#3752,.T.);
#5712=EDGE_CURVE('',#4439,#4439,#3753,.T.);
#5713=EDGE_CURVE('',#4439,#4406,#2866,.T.);
#5714=EDGE_CURVE('',#4433,#4440,#2867,.T.);
#5715=EDGE_CURVE('',#4440,#4440,#3754,.T.);
#5716=EDGE_CURVE('',#4420,#4441,#2868,.T.);
#5717=EDGE_CURVE('',#4441,#4441,#3755,.T.);
#5718=EDGE_CURVE('',#4442,#4443,#2869,.T.);
#5719=EDGE_CURVE('',#4444,#4442,#2870,.T.);
#5720=EDGE_CURVE('',#4445,#4444,#2871,.T.);
#5721=EDGE_CURVE('',#4445,#4443,#2872,.T.);
#5722=EDGE_CURVE('',#4446,#4447,#2873,.T.);
#5723=EDGE_CURVE('',#4446,#4448,#2874,.T.);
#5724=EDGE_CURVE('',#4449,#4448,#2875,.T.);
#5725=EDGE_CURVE('',#4447,#4449,#2876,.T.);
#5726=EDGE_CURVE('',#4450,#4451,#2877,.T.);
#5727=EDGE_CURVE('',#4450,#4452,#2878,.T.);
#5728=EDGE_CURVE('',#4453,#4452,#2879,.T.);
#5729=EDGE_CURVE('',#4451,#4453,#2880,.T.);
#5730=EDGE_CURVE('',#4454,#4455,#2881,.T.);
#5731=EDGE_CURVE('',#4454,#4456,#2882,.T.);
#5732=EDGE_CURVE('',#4457,#4456,#2883,.T.);
#5733=EDGE_CURVE('',#4455,#4457,#2884,.T.);
#5734=EDGE_CURVE('',#4458,#4459,#2885,.T.);
#5735=EDGE_CURVE('',#4458,#4460,#2886,.T.);
#5736=EDGE_CURVE('',#4461,#4460,#2887,.T.);
#5737=EDGE_CURVE('',#4459,#4461,#2888,.T.);
#5738=EDGE_CURVE('',#4462,#4463,#2889,.T.);
#5739=EDGE_CURVE('',#4464,#4462,#2890,.T.);
#5740=EDGE_CURVE('',#4465,#4464,#2891,.T.);
#5741=EDGE_CURVE('',#4465,#4463,#2892,.T.);
#5742=EDGE_CURVE('',#4466,#4467,#2893,.T.);
#5743=EDGE_CURVE('',#4468,#4466,#2894,.T.);
#5744=EDGE_CURVE('',#4469,#4468,#2895,.T.);
#5745=EDGE_CURVE('',#4469,#4467,#2896,.T.);
#5746=EDGE_CURVE('',#4470,#4470,#3756,.T.);
#5747=EDGE_CURVE('',#4471,#4471,#3757,.T.);
#5748=EDGE_CURVE('',#4443,#4458,#2897,.T.);
#5749=EDGE_CURVE('',#4460,#4445,#2898,.T.);
#5750=EDGE_CURVE('',#4463,#4446,#2899,.T.);
#5751=EDGE_CURVE('',#4448,#4465,#2900,.T.);
#5752=EDGE_CURVE('',#4467,#4450,#2901,.T.);
#5753=EDGE_CURVE('',#4452,#4469,#2902,.T.);
#5754=EDGE_CURVE('',#4472,#4454,#2903,.T.);
#5755=EDGE_CURVE('',#4473,#4472,#2904,.T.);
#5756=EDGE_CURVE('',#4456,#4473,#2905,.T.);
#5757=EDGE_CURVE('',#4474,#4472,#2906,.T.);
#5758=EDGE_CURVE('',#4475,#4474,#2907,.T.);
#5759=EDGE_CURVE('',#4473,#4475,#2908,.T.);
#5760=EDGE_CURVE('',#4476,#4477,#2909,.T.);
#5761=EDGE_CURVE('',#4478,#4477,#733,.T.);
#5762=EDGE_CURVE('',#4404,#4478,#734,.T.);
#5763=EDGE_CURVE('',#4476,#4401,#735,.T.);
#5764=EDGE_CURVE('',#4475,#4479,#2910,.T.);
#5765=EDGE_CURVE('',#4400,#4479,#736,.T.);
#5766=EDGE_CURVE('',#4480,#4403,#737,.T.);
#5767=EDGE_CURVE('',#4481,#4480,#738,.T.);
#5768=EDGE_CURVE('',#4481,#4457,#2911,.T.);
#5769=EDGE_CURVE('',#4468,#4482,#2912,.T.);
#5770=EDGE_CURVE('',#4483,#4482,#739,.T.);
#5771=EDGE_CURVE('',#4484,#4483,#740,.T.);
#5772=EDGE_CURVE('',#4485,#4484,#2913,.T.);
#5773=EDGE_CURVE('',#4486,#4485,#741,.T.);
#5774=EDGE_CURVE('',#4487,#4486,#742,.T.);
#5775=EDGE_CURVE('',#4487,#4453,#2914,.T.);
#5776=EDGE_CURVE('',#4464,#4488,#2915,.T.);
#5777=EDGE_CURVE('',#4396,#4488,#743,.T.);
#5778=EDGE_CURVE('',#4489,#4395,#2916,.T.);
#5779=EDGE_CURVE('',#4490,#4489,#744,.T.);
#5780=EDGE_CURVE('',#4491,#4490,#745,.T.);
#5781=EDGE_CURVE('',#4491,#4449,#2917,.T.);
#5782=EDGE_CURVE('',#4492,#4459,#2918,.T.);
#5783=EDGE_CURVE('',#4492,#4493,#746,.T.);
#5784=EDGE_CURVE('',#4493,#4494,#2919,.T.);
#5785=EDGE_CURVE('',#4494,#4495,#747,.T.);
#5786=EDGE_CURVE('',#4442,#4495,#2920,.T.);
#5787=EDGE_CURVE('',#4481,#4477,#748,.T.);
#5788=EDGE_CURVE('',#4476,#4479,#749,.T.);
#5789=EDGE_CURVE('',#4496,#4474,#2921,.T.);
#5790=EDGE_CURVE('',#4496,#4482,#750,.T.);
#5791=EDGE_CURVE('',#4497,#4466,#2922,.T.);
#5792=EDGE_CURVE('',#4497,#4488,#751,.T.);
#5793=EDGE_CURVE('',#4498,#4462,#2923,.T.);
#5794=EDGE_CURVE('',#4498,#4499,#752,.T.);
#5795=EDGE_CURVE('',#4499,#4492,#753,.T.);
#5796=EDGE_CURVE('',#4461,#4500,#2924,.T.);
#5797=EDGE_CURVE('',#4501,#4500,#754,.T.);
#5798=EDGE_CURVE('',#4501,#4502,#755,.T.);
#5799=EDGE_CURVE('',#4503,#4502,#756,.T.);
#5800=EDGE_CURVE('',#4503,#4504,#2925,.T.);
#5801=EDGE_CURVE('',#4505,#4504,#757,.T.);
#5802=EDGE_CURVE('',#4505,#4506,#758,.T.);
#5803=EDGE_CURVE('',#4507,#4506,#759,.T.);
#5804=EDGE_CURVE('',#4507,#4444,#2926,.T.);
#5805=EDGE_CURVE('',#4495,#4508,#760,.T.);
#5806=EDGE_CURVE('',#4508,#4509,#761,.T.);
#5807=EDGE_CURVE('',#4447,#4509,#2927,.T.);
#5808=EDGE_CURVE('',#4491,#4510,#762,.T.);
#5809=EDGE_CURVE('',#4451,#4510,#2928,.T.);
#5810=EDGE_CURVE('',#4487,#4511,#763,.T.);
#5811=EDGE_CURVE('',#4455,#4511,#2929,.T.);
#5812=EDGE_CURVE('',#4512,#4513,#764,.T.);
#5813=EDGE_CURVE('',#4513,#4514,#765,.T.);
#5814=EDGE_CURVE('',#4514,#4515,#2930,.T.);
#5815=EDGE_CURVE('',#4515,#4516,#766,.T.);
#5816=EDGE_CURVE('',#4516,#4517,#767,.T.);
#5817=EDGE_CURVE('',#4512,#4517,#2931,.T.);
#5818=EDGE_CURVE('',#4407,#4471,#2932,.T.);
#5819=EDGE_CURVE('',#4518,#4518,#3758,.T.);
#5820=EDGE_CURVE('',#4518,#4470,#2933,.T.);
#5821=EDGE_CURVE('',#4512,#4519,#768,.T.);
#5822=EDGE_CURVE('',#4520,#4517,#769,.T.);
#5823=EDGE_CURVE('',#4521,#4520,#770,.T.);
#5824=EDGE_CURVE('',#4522,#4521,#2934,.T.);
#5825=EDGE_CURVE('',#4519,#4522,#771,.T.);
#5826=EDGE_CURVE('',#4480,#4478,#772,.T.);
#5827=EDGE_CURVE('',#4519,#4523,#773,.T.);
#5828=EDGE_CURVE('',#4523,#4513,#774,.T.);
#5829=EDGE_CURVE('',#4524,#4522,#775,.T.);
#5830=EDGE_CURVE('',#4523,#4524,#3759,.F.);
#5831=EDGE_CURVE('',#4521,#4525,#776,.T.);
#5832=EDGE_CURVE('',#4525,#4524,#2935,.T.);
#5833=EDGE_CURVE('',#4516,#4526,#777,.T.);
#5834=EDGE_CURVE('',#4526,#4520,#778,.T.);
#5835=EDGE_CURVE('',#4527,#4511,#779,.T.);
#5836=EDGE_CURVE('',#4528,#4527,#780,.T.);
#5837=EDGE_CURVE('',#4529,#4528,#2936,.T.);
#5838=EDGE_CURVE('',#4530,#4529,#781,.T.);
#5839=EDGE_CURVE('',#4496,#4530,#782,.T.);
#5840=EDGE_CURVE('',#4486,#4527,#783,.T.);
#5841=EDGE_CURVE('',#4528,#4485,#784,.T.);
#5842=EDGE_CURVE('',#4484,#4529,#785,.T.);
#5843=EDGE_CURVE('',#4530,#4483,#786,.T.);
#5844=EDGE_CURVE('',#4531,#4510,#787,.T.);
#5845=EDGE_CURVE('',#4532,#4531,#788,.T.);
#5846=EDGE_CURVE('',#4398,#4532,#2937,.T.);
#5847=EDGE_CURVE('',#4497,#4397,#789,.T.);
#5848=EDGE_CURVE('',#4490,#4531,#790,.T.);
#5849=EDGE_CURVE('',#4532,#4392,#791,.T.);
#5850=EDGE_CURVE('',#4391,#4489,#792,.T.);
#5851=EDGE_CURVE('',#4533,#4509,#793,.T.);
#5852=EDGE_CURVE('',#4534,#4533,#794,.T.);
#5853=EDGE_CURVE('',#4535,#4534,#2938,.T.);
#5854=EDGE_CURVE('',#4536,#4535,#795,.T.);
#5855=EDGE_CURVE('',#4498,#4536,#796,.T.);
#5856=EDGE_CURVE('',#4508,#4537,#797,.T.);
#5857=EDGE_CURVE('',#4537,#4533,#798,.T.);
#5858=EDGE_CURVE('',#4538,#4537,#3760,.F.);
#5859=EDGE_CURVE('',#4534,#4538,#799,.T.);
#5860=EDGE_CURVE('',#4538,#4539,#2939,.T.);
#5861=EDGE_CURVE('',#4539,#4535,#800,.T.);
#5862=EDGE_CURVE('',#4536,#4540,#801,.T.);
#5863=EDGE_CURVE('',#4540,#4499,#802,.T.);
#5864=EDGE_CURVE('',#4540,#4539,#3761,.F.);
#5865=EDGE_CURVE('',#4539,#4493,#3762,.F.);
#5866=EDGE_CURVE('',#4493,#4540,#3763,.F.);
#5867=EDGE_CURVE('',#4525,#4526,#3764,.F.);
#5868=EDGE_CURVE('',#4526,#4541,#3765,.F.);
#5869=EDGE_CURVE('',#4541,#4525,#3766,.F.);
#5870=EDGE_CURVE('',#4537,#4494,#3767,.F.);
#5871=EDGE_CURVE('',#4494,#4538,#3768,.F.);
#5872=EDGE_CURVE('',#4542,#4523,#3769,.F.);
#5873=EDGE_CURVE('',#4524,#4542,#3770,.F.);
#5874=EDGE_CURVE('',#4542,#4541,#2940,.T.);
#5875=EDGE_CURVE('',#4514,#4542,#803,.T.);
#5876=EDGE_CURVE('',#4541,#4515,#804,.T.);
#5877=EDGE_CURVE('',#4543,#4544,#3771,.F.);
#5878=EDGE_CURVE('',#4545,#4543,#3772,.F.);
#5879=EDGE_CURVE('',#4544,#4545,#3773,.F.);
#5880=EDGE_CURVE('',#4546,#4547,#3774,.F.);
#5881=EDGE_CURVE('',#4548,#4546,#3775,.F.);
#5882=EDGE_CURVE('',#4547,#4548,#3776,.F.);
#5883=EDGE_CURVE('',#4549,#4550,#3777,.F.);
#5884=EDGE_CURVE('',#4551,#4549,#3778,.F.);
#5885=EDGE_CURVE('',#4550,#4551,#3779,.F.);
#5886=EDGE_CURVE('',#4544,#4551,#2941,.T.);
#5887=EDGE_CURVE('',#4549,#4543,#2942,.T.);
#5888=EDGE_CURVE('',#4506,#4550,#805,.T.);
#5889=EDGE_CURVE('',#4551,#4507,#806,.T.);
#5890=EDGE_CURVE('',#4552,#4553,#3780,.F.);
#5891=EDGE_CURVE('',#4554,#4552,#3781,.F.);
#5892=EDGE_CURVE('',#4553,#4554,#3782,.F.);
#5893=EDGE_CURVE('',#4552,#4548,#2943,.T.);
#5894=EDGE_CURVE('',#4546,#4554,#2944,.T.);
#5895=EDGE_CURVE('',#4550,#4553,#807,.T.);
#5896=EDGE_CURVE('',#4554,#4549,#808,.T.);
#5897=EDGE_CURVE('',#4504,#4552,#809,.T.);
#5898=EDGE_CURVE('',#4553,#4505,#810,.T.);
#5899=EDGE_CURVE('',#4502,#4547,#811,.T.);
#5900=EDGE_CURVE('',#4548,#4503,#812,.T.);
#5901=EDGE_CURVE('',#4547,#4545,#813,.T.);
#5902=EDGE_CURVE('',#4543,#4546,#814,.T.);
#5903=EDGE_CURVE('',#4500,#4544,#815,.T.);
#5904=EDGE_CURVE('',#4545,#4501,#816,.T.);
#7965=ORIENTED_EDGE('',*,*,#5641,.F.);
#7966=ORIENTED_EDGE('',*,*,#5642,.T.);
#7967=ORIENTED_EDGE('',*,*,#5643,.F.);
#7968=ORIENTED_EDGE('',*,*,#5644,.T.);
#7969=ORIENTED_EDGE('',*,*,#5645,.F.);
#7970=ORIENTED_EDGE('',*,*,#5646,.T.);
#7971=ORIENTED_EDGE('',*,*,#5647,.F.);
#7972=ORIENTED_EDGE('',*,*,#5648,.T.);
#7973=ORIENTED_EDGE('',*,*,#5643,.T.);
#7974=ORIENTED_EDGE('',*,*,#5649,.F.);
#7975=ORIENTED_EDGE('',*,*,#5650,.T.);
#7976=ORIENTED_EDGE('',*,*,#5651,.F.);
#7977=ORIENTED_EDGE('',*,*,#5652,.T.);
#7978=ORIENTED_EDGE('',*,*,#5653,.F.);
#7979=ORIENTED_EDGE('',*,*,#5647,.T.);
#7980=ORIENTED_EDGE('',*,*,#5654,.F.);
#7981=ORIENTED_EDGE('',*,*,#5655,.T.);
#7982=ORIENTED_EDGE('',*,*,#5656,.F.);
#7983=ORIENTED_EDGE('',*,*,#5657,.T.);
#7984=ORIENTED_EDGE('',*,*,#5658,.F.);
#7985=ORIENTED_EDGE('',*,*,#5659,.T.);
#7986=ORIENTED_EDGE('',*,*,#5660,.T.);
#7987=ORIENTED_EDGE('',*,*,#5654,.T.);
#7988=ORIENTED_EDGE('',*,*,#5648,.F.);
#7989=ORIENTED_EDGE('',*,*,#5658,.T.);
#7990=ORIENTED_EDGE('',*,*,#5661,.T.);
#7991=ORIENTED_EDGE('',*,*,#5662,.T.);
#7992=ORIENTED_EDGE('',*,*,#5642,.F.);
#7993=ORIENTED_EDGE('',*,*,#5663,.T.);
#7994=ORIENTED_EDGE('',*,*,#5664,.T.);
#7995=ORIENTED_EDGE('',*,*,#5665,.T.);
#7996=ORIENTED_EDGE('',*,*,#5666,.F.);
#7997=ORIENTED_EDGE('',*,*,#5667,.T.);
#7998=ORIENTED_EDGE('',*,*,#5668,.T.);
#7999=ORIENTED_EDGE('',*,*,#5669,.F.);
#8000=ORIENTED_EDGE('',*,*,#5670,.F.);
#8001=ORIENTED_EDGE('',*,*,#5671,.T.);
#8002=ORIENTED_EDGE('',*,*,#5672,.T.);
#8003=ORIENTED_EDGE('',*,*,#5667,.F.);
#8004=ORIENTED_EDGE('',*,*,#5673,.F.);
#8005=ORIENTED_EDGE('',*,*,#5674,.T.);
#8006=ORIENTED_EDGE('',*,*,#5675,.T.);
#8007=ORIENTED_EDGE('',*,*,#5671,.F.);
#8008=ORIENTED_EDGE('',*,*,#5676,.F.);
#8009=ORIENTED_EDGE('',*,*,#5677,.T.);
#8010=ORIENTED_EDGE('',*,*,#5678,.T.);
#8011=ORIENTED_EDGE('',*,*,#5674,.F.);
#8012=ORIENTED_EDGE('',*,*,#5679,.F.);
#8013=ORIENTED_EDGE('',*,*,#5680,.T.);
#8014=ORIENTED_EDGE('',*,*,#5681,.T.);
#8015=ORIENTED_EDGE('',*,*,#5677,.F.);
#8016=ORIENTED_EDGE('',*,*,#5682,.F.);
#8017=ORIENTED_EDGE('',*,*,#5669,.T.);
#8018=ORIENTED_EDGE('',*,*,#5683,.T.);
#8019=ORIENTED_EDGE('',*,*,#5680,.F.);
#8020=ORIENTED_EDGE('',*,*,#5683,.F.);
#8021=ORIENTED_EDGE('',*,*,#5668,.F.);
#8022=ORIENTED_EDGE('',*,*,#5672,.F.);
#8023=ORIENTED_EDGE('',*,*,#5675,.F.);
#8024=ORIENTED_EDGE('',*,*,#5678,.F.);
#8025=ORIENTED_EDGE('',*,*,#5681,.F.);
#8026=ORIENTED_EDGE('',*,*,#5684,.F.);
#8027=ORIENTED_EDGE('',*,*,#5685,.F.);
#8028=ORIENTED_EDGE('',*,*,#5686,.T.);
#8029=ORIENTED_EDGE('',*,*,#5687,.T.);
#8030=ORIENTED_EDGE('',*,*,#5688,.F.);
#8031=ORIENTED_EDGE('',*,*,#5689,.F.);
#8032=ORIENTED_EDGE('',*,*,#5690,.T.);
#8033=ORIENTED_EDGE('',*,*,#5691,.T.);
#8034=ORIENTED_EDGE('',*,*,#5686,.F.);
#8035=ORIENTED_EDGE('',*,*,#5692,.F.);
#8036=ORIENTED_EDGE('',*,*,#5693,.T.);
#8037=ORIENTED_EDGE('',*,*,#5694,.T.);
#8038=ORIENTED_EDGE('',*,*,#5690,.F.);
#8039=ORIENTED_EDGE('',*,*,#5695,.F.);
#8040=ORIENTED_EDGE('',*,*,#5696,.T.);
#8041=ORIENTED_EDGE('',*,*,#5697,.T.);
#8042=ORIENTED_EDGE('',*,*,#5693,.F.);
#8043=ORIENTED_EDGE('',*,*,#5698,.F.);
#8044=ORIENTED_EDGE('',*,*,#5699,.T.);
#8045=ORIENTED_EDGE('',*,*,#5700,.T.);
#8046=ORIENTED_EDGE('',*,*,#5696,.F.);
#8047=ORIENTED_EDGE('',*,*,#5701,.F.);
#8048=ORIENTED_EDGE('',*,*,#5688,.T.);
#8049=ORIENTED_EDGE('',*,*,#5702,.T.);
#8050=ORIENTED_EDGE('',*,*,#5699,.F.);
#8051=ORIENTED_EDGE('',*,*,#5702,.F.);
#8052=ORIENTED_EDGE('',*,*,#5687,.F.);
#8053=ORIENTED_EDGE('',*,*,#5691,.F.);
#8054=ORIENTED_EDGE('',*,*,#5694,.F.);
#8055=ORIENTED_EDGE('',*,*,#5697,.F.);
#8056=ORIENTED_EDGE('',*,*,#5700,.F.);
#8057=ORIENTED_EDGE('',*,*,#5703,.F.);
#8058=ORIENTED_EDGE('',*,*,#5704,.F.);
#8059=ORIENTED_EDGE('',*,*,#5705,.T.);
#8060=ORIENTED_EDGE('',*,*,#5663,.F.);
#8061=ORIENTED_EDGE('',*,*,#5705,.F.);
#8062=ORIENTED_EDGE('',*,*,#5706,.F.);
#8063=ORIENTED_EDGE('',*,*,#5707,.T.);
#8064=ORIENTED_EDGE('',*,*,#5708,.F.);
#8065=ORIENTED_EDGE('',*,*,#5707,.F.);
#8066=ORIENTED_EDGE('',*,*,#5709,.F.);
#8067=ORIENTED_EDGE('',*,*,#5710,.T.);
#8068=ORIENTED_EDGE('',*,*,#5711,.F.);
#8069=ORIENTED_EDGE('',*,*,#5710,.F.);
#8070=ORIENTED_EDGE('',*,*,#5712,.F.);
#8071=ORIENTED_EDGE('',*,*,#5713,.T.);
#8072=ORIENTED_EDGE('',*,*,#5664,.F.);
#8073=ORIENTED_EDGE('',*,*,#5713,.F.);
#8074=ORIENTED_EDGE('',*,*,#5703,.T.);
#8075=ORIENTED_EDGE('',*,*,#5714,.T.);
#8076=ORIENTED_EDGE('',*,*,#5715,.F.);
#8077=ORIENTED_EDGE('',*,*,#5714,.F.);
#8078=ORIENTED_EDGE('',*,*,#5684,.T.);
#8079=ORIENTED_EDGE('',*,*,#5716,.T.);
#8080=ORIENTED_EDGE('',*,*,#5717,.F.);
#8081=ORIENTED_EDGE('',*,*,#5716,.F.);
#8082=ORIENTED_EDGE('',*,*,#5718,.F.);
#8083=ORIENTED_EDGE('',*,*,#5719,.F.);
#8084=ORIENTED_EDGE('',*,*,#5720,.F.);
#8085=ORIENTED_EDGE('',*,*,#5721,.T.);
#8086=ORIENTED_EDGE('',*,*,#5722,.F.);
#8087=ORIENTED_EDGE('',*,*,#5723,.T.);
#8088=ORIENTED_EDGE('',*,*,#5724,.F.);
#8089=ORIENTED_EDGE('',*,*,#5725,.F.);
#8090=ORIENTED_EDGE('',*,*,#5726,.F.);
#8091=ORIENTED_EDGE('',*,*,#5727,.T.);
#8092=ORIENTED_EDGE('',*,*,#5728,.F.);
#8093=ORIENTED_EDGE('',*,*,#5729,.F.);
#8094=ORIENTED_EDGE('',*,*,#5730,.F.);
#8095=ORIENTED_EDGE('',*,*,#5731,.T.);
#8096=ORIENTED_EDGE('',*,*,#5732,.F.);
#8097=ORIENTED_EDGE('',*,*,#5733,.F.);
#8098=ORIENTED_EDGE('',*,*,#5734,.F.);
#8099=ORIENTED_EDGE('',*,*,#5735,.T.);
#8100=ORIENTED_EDGE('',*,*,#5736,.F.);
#8101=ORIENTED_EDGE('',*,*,#5737,.F.);
#8102=ORIENTED_EDGE('',*,*,#5738,.F.);
#8103=ORIENTED_EDGE('',*,*,#5739,.F.);
#8104=ORIENTED_EDGE('',*,*,#5740,.F.);
#8105=ORIENTED_EDGE('',*,*,#5741,.T.);
#8106=ORIENTED_EDGE('',*,*,#5742,.F.);
#8107=ORIENTED_EDGE('',*,*,#5743,.F.);
#8108=ORIENTED_EDGE('',*,*,#5744,.F.);
#8109=ORIENTED_EDGE('',*,*,#5745,.T.);
#8110=ORIENTED_EDGE('',*,*,#5746,.F.);
#8111=ORIENTED_EDGE('',*,*,#5715,.T.);
#8112=ORIENTED_EDGE('',*,*,#5747,.F.);
#8113=ORIENTED_EDGE('',*,*,#5717,.T.);
#8114=ORIENTED_EDGE('',*,*,#5748,.F.);
#8115=ORIENTED_EDGE('',*,*,#5721,.F.);
#8116=ORIENTED_EDGE('',*,*,#5749,.F.);
#8117=ORIENTED_EDGE('',*,*,#5735,.F.);
#8118=ORIENTED_EDGE('',*,*,#5750,.F.);
#8119=ORIENTED_EDGE('',*,*,#5741,.F.);
#8120=ORIENTED_EDGE('',*,*,#5751,.F.);
#8121=ORIENTED_EDGE('',*,*,#5723,.F.);
#8122=ORIENTED_EDGE('',*,*,#5752,.F.);
#8123=ORIENTED_EDGE('',*,*,#5745,.F.);
#8124=ORIENTED_EDGE('',*,*,#5753,.F.);
#8125=ORIENTED_EDGE('',*,*,#5727,.F.);
#8126=ORIENTED_EDGE('',*,*,#5754,.F.);
#8127=ORIENTED_EDGE('',*,*,#5755,.F.);
#8128=ORIENTED_EDGE('',*,*,#5756,.F.);
#8129=ORIENTED_EDGE('',*,*,#5731,.F.);
#8130=ORIENTED_EDGE('',*,*,#5757,.F.);
#8131=ORIENTED_EDGE('',*,*,#5758,.F.);
#8132=ORIENTED_EDGE('',*,*,#5759,.F.);
#8133=ORIENTED_EDGE('',*,*,#5755,.T.);
#8134=ORIENTED_EDGE('',*,*,#5760,.T.);
#8135=ORIENTED_EDGE('',*,*,#5761,.F.);
#8136=ORIENTED_EDGE('',*,*,#5762,.F.);
#8137=ORIENTED_EDGE('',*,*,#5661,.F.);
#8138=ORIENTED_EDGE('',*,*,#5657,.F.);
#8139=ORIENTED_EDGE('',*,*,#5763,.F.);
#8140=ORIENTED_EDGE('',*,*,#5732,.T.);
#8141=ORIENTED_EDGE('',*,*,#5756,.T.);
#8142=ORIENTED_EDGE('',*,*,#5759,.T.);
#8143=ORIENTED_EDGE('',*,*,#5764,.T.);
#8144=ORIENTED_EDGE('',*,*,#5765,.F.);
#8145=ORIENTED_EDGE('',*,*,#5655,.F.);
#8146=ORIENTED_EDGE('',*,*,#5660,.F.);
#8147=ORIENTED_EDGE('',*,*,#5766,.F.);
#8148=ORIENTED_EDGE('',*,*,#5767,.F.);
#8149=ORIENTED_EDGE('',*,*,#5768,.T.);
#8150=ORIENTED_EDGE('',*,*,#5728,.T.);
#8151=ORIENTED_EDGE('',*,*,#5753,.T.);
#8152=ORIENTED_EDGE('',*,*,#5744,.T.);
#8153=ORIENTED_EDGE('',*,*,#5769,.T.);
#8154=ORIENTED_EDGE('',*,*,#5770,.F.);
#8155=ORIENTED_EDGE('',*,*,#5771,.F.);
#8156=ORIENTED_EDGE('',*,*,#5772,.F.);
#8157=ORIENTED_EDGE('',*,*,#5773,.F.);
#8158=ORIENTED_EDGE('',*,*,#5774,.F.);
#8159=ORIENTED_EDGE('',*,*,#5775,.T.);
#8160=ORIENTED_EDGE('',*,*,#5724,.T.);
#8161=ORIENTED_EDGE('',*,*,#5751,.T.);
#8162=ORIENTED_EDGE('',*,*,#5740,.T.);
#8163=ORIENTED_EDGE('',*,*,#5776,.T.);
#8164=ORIENTED_EDGE('',*,*,#5777,.F.);
#8165=ORIENTED_EDGE('',*,*,#5650,.F.);
#8166=ORIENTED_EDGE('',*,*,#5778,.F.);
#8167=ORIENTED_EDGE('',*,*,#5779,.F.);
#8168=ORIENTED_EDGE('',*,*,#5780,.F.);
#8169=ORIENTED_EDGE('',*,*,#5781,.T.);
#8170=ORIENTED_EDGE('',*,*,#5718,.T.);
#8171=ORIENTED_EDGE('',*,*,#5748,.T.);
#8172=ORIENTED_EDGE('',*,*,#5734,.T.);
#8173=ORIENTED_EDGE('',*,*,#5782,.F.);
#8174=ORIENTED_EDGE('',*,*,#5783,.T.);
#8175=ORIENTED_EDGE('',*,*,#5784,.T.);
#8176=ORIENTED_EDGE('',*,*,#5785,.T.);
#8177=ORIENTED_EDGE('',*,*,#5786,.F.);
#8178=ORIENTED_EDGE('',*,*,#5733,.T.);
#8179=ORIENTED_EDGE('',*,*,#5768,.F.);
#8180=ORIENTED_EDGE('',*,*,#5787,.T.);
#8181=ORIENTED_EDGE('',*,*,#5760,.F.);
#8182=ORIENTED_EDGE('',*,*,#5788,.T.);
#8183=ORIENTED_EDGE('',*,*,#5764,.F.);
#8184=ORIENTED_EDGE('',*,*,#5758,.T.);
#8185=ORIENTED_EDGE('',*,*,#5789,.F.);
#8186=ORIENTED_EDGE('',*,*,#5790,.T.);
#8187=ORIENTED_EDGE('',*,*,#5769,.F.);
#8188=ORIENTED_EDGE('',*,*,#5743,.T.);
#8189=ORIENTED_EDGE('',*,*,#5791,.F.);
#8190=ORIENTED_EDGE('',*,*,#5792,.T.);
#8191=ORIENTED_EDGE('',*,*,#5776,.F.);
#8192=ORIENTED_EDGE('',*,*,#5739,.T.);
#8193=ORIENTED_EDGE('',*,*,#5793,.F.);
#8194=ORIENTED_EDGE('',*,*,#5794,.T.);
#8195=ORIENTED_EDGE('',*,*,#5795,.T.);
#8196=ORIENTED_EDGE('',*,*,#5782,.T.);
#8197=ORIENTED_EDGE('',*,*,#5737,.T.);
#8198=ORIENTED_EDGE('',*,*,#5796,.T.);
#8199=ORIENTED_EDGE('',*,*,#5797,.F.);
#8200=ORIENTED_EDGE('',*,*,#5798,.T.);
#8201=ORIENTED_EDGE('',*,*,#5799,.F.);
#8202=ORIENTED_EDGE('',*,*,#5800,.T.);
#8203=ORIENTED_EDGE('',*,*,#5801,.F.);
#8204=ORIENTED_EDGE('',*,*,#5802,.T.);
#8205=ORIENTED_EDGE('',*,*,#5803,.F.);
#8206=ORIENTED_EDGE('',*,*,#5804,.T.);
#8207=ORIENTED_EDGE('',*,*,#5719,.T.);
#8208=ORIENTED_EDGE('',*,*,#5786,.T.);
#8209=ORIENTED_EDGE('',*,*,#5805,.T.);
#8210=ORIENTED_EDGE('',*,*,#5806,.T.);
#8211=ORIENTED_EDGE('',*,*,#5807,.F.);
#8212=ORIENTED_EDGE('',*,*,#5725,.T.);
#8213=ORIENTED_EDGE('',*,*,#5781,.F.);
#8214=ORIENTED_EDGE('',*,*,#5808,.T.);
#8215=ORIENTED_EDGE('',*,*,#5809,.F.);
#8216=ORIENTED_EDGE('',*,*,#5729,.T.);
#8217=ORIENTED_EDGE('',*,*,#5775,.F.);
#8218=ORIENTED_EDGE('',*,*,#5810,.T.);
#8219=ORIENTED_EDGE('',*,*,#5811,.F.);
#8220=ORIENTED_EDGE('',*,*,#5812,.T.);
#8221=ORIENTED_EDGE('',*,*,#5813,.T.);
#8222=ORIENTED_EDGE('',*,*,#5814,.T.);
#8223=ORIENTED_EDGE('',*,*,#5815,.T.);
#8224=ORIENTED_EDGE('',*,*,#5816,.T.);
#8225=ORIENTED_EDGE('',*,*,#5817,.F.);
#8226=ORIENTED_EDGE('',*,*,#5665,.F.);
#8227=ORIENTED_EDGE('',*,*,#5818,.T.);
#8228=ORIENTED_EDGE('',*,*,#5747,.T.);
#8229=ORIENTED_EDGE('',*,*,#5818,.F.);
#8230=ORIENTED_EDGE('',*,*,#5819,.F.);
#8231=ORIENTED_EDGE('',*,*,#5820,.T.);
#8232=ORIENTED_EDGE('',*,*,#5746,.T.);
#8233=ORIENTED_EDGE('',*,*,#5820,.F.);
#8234=ORIENTED_EDGE('',*,*,#5821,.F.);
#8235=ORIENTED_EDGE('',*,*,#5817,.T.);
#8236=ORIENTED_EDGE('',*,*,#5822,.F.);
#8237=ORIENTED_EDGE('',*,*,#5823,.F.);
#8238=ORIENTED_EDGE('',*,*,#5824,.F.);
#8239=ORIENTED_EDGE('',*,*,#5825,.F.);
#8240=ORIENTED_EDGE('',*,*,#5761,.T.);
#8241=ORIENTED_EDGE('',*,*,#5787,.F.);
#8242=ORIENTED_EDGE('',*,*,#5767,.T.);
#8243=ORIENTED_EDGE('',*,*,#5826,.T.);
#8244=ORIENTED_EDGE('',*,*,#5821,.T.);
#8245=ORIENTED_EDGE('',*,*,#5827,.T.);
#8246=ORIENTED_EDGE('',*,*,#5828,.T.);
#8247=ORIENTED_EDGE('',*,*,#5812,.F.);
#8248=ORIENTED_EDGE('',*,*,#5641,.T.);
#8249=ORIENTED_EDGE('',*,*,#5662,.F.);
#8250=ORIENTED_EDGE('',*,*,#5762,.T.);
#8251=ORIENTED_EDGE('',*,*,#5826,.F.);
#8252=ORIENTED_EDGE('',*,*,#5766,.T.);
#8253=ORIENTED_EDGE('',*,*,#5659,.F.);
#8254=ORIENTED_EDGE('',*,*,#5825,.T.);
#8255=ORIENTED_EDGE('',*,*,#5829,.F.);
#8256=ORIENTED_EDGE('',*,*,#5830,.F.);
#8257=ORIENTED_EDGE('',*,*,#5827,.F.);
#8258=ORIENTED_EDGE('',*,*,#5824,.T.);
#8259=ORIENTED_EDGE('',*,*,#5831,.T.);
#8260=ORIENTED_EDGE('',*,*,#5832,.T.);
#8261=ORIENTED_EDGE('',*,*,#5829,.T.);
#8262=ORIENTED_EDGE('',*,*,#5763,.T.);
#8263=ORIENTED_EDGE('',*,*,#5656,.T.);
#8264=ORIENTED_EDGE('',*,*,#5765,.T.);
#8265=ORIENTED_EDGE('',*,*,#5788,.F.);
#8266=ORIENTED_EDGE('',*,*,#5822,.T.);
#8267=ORIENTED_EDGE('',*,*,#5816,.F.);
#8268=ORIENTED_EDGE('',*,*,#5833,.T.);
#8269=ORIENTED_EDGE('',*,*,#5834,.T.);
#8270=ORIENTED_EDGE('',*,*,#5730,.T.);
#8271=ORIENTED_EDGE('',*,*,#5811,.T.);
#8272=ORIENTED_EDGE('',*,*,#5835,.F.);
#8273=ORIENTED_EDGE('',*,*,#5836,.F.);
#8274=ORIENTED_EDGE('',*,*,#5837,.F.);
#8275=ORIENTED_EDGE('',*,*,#5838,.F.);
#8276=ORIENTED_EDGE('',*,*,#5839,.F.);
#8277=ORIENTED_EDGE('',*,*,#5789,.T.);
#8278=ORIENTED_EDGE('',*,*,#5757,.T.);
#8279=ORIENTED_EDGE('',*,*,#5754,.T.);
#8280=ORIENTED_EDGE('',*,*,#5835,.T.);
#8281=ORIENTED_EDGE('',*,*,#5810,.F.);
#8282=ORIENTED_EDGE('',*,*,#5774,.T.);
#8283=ORIENTED_EDGE('',*,*,#5840,.T.);
#8284=ORIENTED_EDGE('',*,*,#5836,.T.);
#8285=ORIENTED_EDGE('',*,*,#5840,.F.);
#8286=ORIENTED_EDGE('',*,*,#5773,.T.);
#8287=ORIENTED_EDGE('',*,*,#5841,.F.);
#8288=ORIENTED_EDGE('',*,*,#5837,.T.);
#8289=ORIENTED_EDGE('',*,*,#5841,.T.);
#8290=ORIENTED_EDGE('',*,*,#5772,.T.);
#8291=ORIENTED_EDGE('',*,*,#5842,.T.);
#8292=ORIENTED_EDGE('',*,*,#5838,.T.);
#8293=ORIENTED_EDGE('',*,*,#5842,.F.);
#8294=ORIENTED_EDGE('',*,*,#5771,.T.);
#8295=ORIENTED_EDGE('',*,*,#5843,.F.);
#8296=ORIENTED_EDGE('',*,*,#5839,.T.);
#8297=ORIENTED_EDGE('',*,*,#5843,.T.);
#8298=ORIENTED_EDGE('',*,*,#5770,.T.);
#8299=ORIENTED_EDGE('',*,*,#5790,.F.);
#8300=ORIENTED_EDGE('',*,*,#5726,.T.);
#8301=ORIENTED_EDGE('',*,*,#5809,.T.);
#8302=ORIENTED_EDGE('',*,*,#5844,.F.);
#8303=ORIENTED_EDGE('',*,*,#5845,.F.);
#8304=ORIENTED_EDGE('',*,*,#5846,.F.);
#8305=ORIENTED_EDGE('',*,*,#5652,.F.);
#8306=ORIENTED_EDGE('',*,*,#5847,.F.);
#8307=ORIENTED_EDGE('',*,*,#5791,.T.);
#8308=ORIENTED_EDGE('',*,*,#5742,.T.);
#8309=ORIENTED_EDGE('',*,*,#5752,.T.);
#8310=ORIENTED_EDGE('',*,*,#5844,.T.);
#8311=ORIENTED_EDGE('',*,*,#5808,.F.);
#8312=ORIENTED_EDGE('',*,*,#5780,.T.);
#8313=ORIENTED_EDGE('',*,*,#5848,.T.);
#8314=ORIENTED_EDGE('',*,*,#5645,.T.);
#8315=ORIENTED_EDGE('',*,*,#5849,.F.);
#8316=ORIENTED_EDGE('',*,*,#5845,.T.);
#8317=ORIENTED_EDGE('',*,*,#5848,.F.);
#8318=ORIENTED_EDGE('',*,*,#5779,.T.);
#8319=ORIENTED_EDGE('',*,*,#5850,.F.);
#8320=ORIENTED_EDGE('',*,*,#5653,.T.);
#8321=ORIENTED_EDGE('',*,*,#5846,.T.);
#8322=ORIENTED_EDGE('',*,*,#5849,.T.);
#8323=ORIENTED_EDGE('',*,*,#5646,.F.);
#8324=ORIENTED_EDGE('',*,*,#5850,.T.);
#8325=ORIENTED_EDGE('',*,*,#5778,.T.);
#8326=ORIENTED_EDGE('',*,*,#5649,.T.);
#8327=ORIENTED_EDGE('',*,*,#5644,.F.);
#8328=ORIENTED_EDGE('',*,*,#5711,.T.);
#8329=ORIENTED_EDGE('',*,*,#5708,.T.);
#8330=ORIENTED_EDGE('',*,*,#5819,.T.);
#8331=ORIENTED_EDGE('',*,*,#5847,.T.);
#8332=ORIENTED_EDGE('',*,*,#5651,.T.);
#8333=ORIENTED_EDGE('',*,*,#5777,.T.);
#8334=ORIENTED_EDGE('',*,*,#5792,.F.);
#8335=ORIENTED_EDGE('',*,*,#5722,.T.);
#8336=ORIENTED_EDGE('',*,*,#5807,.T.);
#8337=ORIENTED_EDGE('',*,*,#5851,.F.);
#8338=ORIENTED_EDGE('',*,*,#5852,.F.);
#8339=ORIENTED_EDGE('',*,*,#5853,.F.);
#8340=ORIENTED_EDGE('',*,*,#5854,.F.);
#8341=ORIENTED_EDGE('',*,*,#5855,.F.);
#8342=ORIENTED_EDGE('',*,*,#5793,.T.);
#8343=ORIENTED_EDGE('',*,*,#5738,.T.);
#8344=ORIENTED_EDGE('',*,*,#5750,.T.);
#8345=ORIENTED_EDGE('',*,*,#5851,.T.);
#8346=ORIENTED_EDGE('',*,*,#5806,.F.);
#8347=ORIENTED_EDGE('',*,*,#5856,.T.);
#8348=ORIENTED_EDGE('',*,*,#5857,.T.);
#8349=ORIENTED_EDGE('',*,*,#5852,.T.);
#8350=ORIENTED_EDGE('',*,*,#5857,.F.);
#8351=ORIENTED_EDGE('',*,*,#5858,.F.);
#8352=ORIENTED_EDGE('',*,*,#5859,.F.);
#8353=ORIENTED_EDGE('',*,*,#5853,.T.);
#8354=ORIENTED_EDGE('',*,*,#5859,.T.);
#8355=ORIENTED_EDGE('',*,*,#5860,.T.);
#8356=ORIENTED_EDGE('',*,*,#5861,.T.);
#8357=ORIENTED_EDGE('',*,*,#5855,.T.);
#8358=ORIENTED_EDGE('',*,*,#5862,.T.);
#8359=ORIENTED_EDGE('',*,*,#5863,.T.);
#8360=ORIENTED_EDGE('',*,*,#5794,.F.);
#8361=ORIENTED_EDGE('',*,*,#5854,.T.);
#8362=ORIENTED_EDGE('',*,*,#5861,.F.);
#8363=ORIENTED_EDGE('',*,*,#5864,.F.);
#8364=ORIENTED_EDGE('',*,*,#5862,.F.);
#8365=ORIENTED_EDGE('',*,*,#5865,.T.);
#8366=ORIENTED_EDGE('',*,*,#5866,.T.);
#8367=ORIENTED_EDGE('',*,*,#5864,.T.);
#8368=ORIENTED_EDGE('',*,*,#5867,.T.);
#8369=ORIENTED_EDGE('',*,*,#5868,.T.);
#8370=ORIENTED_EDGE('',*,*,#5869,.T.);
#8371=ORIENTED_EDGE('',*,*,#5858,.T.);
#8372=ORIENTED_EDGE('',*,*,#5870,.T.);
#8373=ORIENTED_EDGE('',*,*,#5871,.T.);
#8374=ORIENTED_EDGE('',*,*,#5865,.F.);
#8375=ORIENTED_EDGE('',*,*,#5860,.F.);
#8376=ORIENTED_EDGE('',*,*,#5871,.F.);
#8377=ORIENTED_EDGE('',*,*,#5784,.F.);
#8378=ORIENTED_EDGE('',*,*,#5805,.F.);
#8379=ORIENTED_EDGE('',*,*,#5785,.F.);
#8380=ORIENTED_EDGE('',*,*,#5870,.F.);
#8381=ORIENTED_EDGE('',*,*,#5856,.F.);
#8382=ORIENTED_EDGE('',*,*,#5872,.T.);
#8383=ORIENTED_EDGE('',*,*,#5830,.T.);
#8384=ORIENTED_EDGE('',*,*,#5873,.T.);
#8385=ORIENTED_EDGE('',*,*,#5873,.F.);
#8386=ORIENTED_EDGE('',*,*,#5832,.F.);
#8387=ORIENTED_EDGE('',*,*,#5869,.F.);
#8388=ORIENTED_EDGE('',*,*,#5874,.F.);
#8389=ORIENTED_EDGE('',*,*,#5813,.F.);
#8390=ORIENTED_EDGE('',*,*,#5828,.F.);
#8391=ORIENTED_EDGE('',*,*,#5872,.F.);
#8392=ORIENTED_EDGE('',*,*,#5875,.F.);
#8393=ORIENTED_EDGE('',*,*,#5815,.F.);
#8394=ORIENTED_EDGE('',*,*,#5876,.F.);
#8395=ORIENTED_EDGE('',*,*,#5868,.F.);
#8396=ORIENTED_EDGE('',*,*,#5833,.F.);
#8397=ORIENTED_EDGE('',*,*,#5823,.T.);
#8398=ORIENTED_EDGE('',*,*,#5834,.F.);
#8399=ORIENTED_EDGE('',*,*,#5867,.F.);
#8400=ORIENTED_EDGE('',*,*,#5831,.F.);
#8401=ORIENTED_EDGE('',*,*,#5795,.F.);
#8402=ORIENTED_EDGE('',*,*,#5863,.F.);
#8403=ORIENTED_EDGE('',*,*,#5866,.F.);
#8404=ORIENTED_EDGE('',*,*,#5783,.F.);
#8405=ORIENTED_EDGE('',*,*,#5875,.T.);
#8406=ORIENTED_EDGE('',*,*,#5874,.T.);
#8407=ORIENTED_EDGE('',*,*,#5876,.T.);
#8408=ORIENTED_EDGE('',*,*,#5814,.F.);
#8409=ORIENTED_EDGE('',*,*,#5877,.F.);
#8410=ORIENTED_EDGE('',*,*,#5878,.F.);
#8411=ORIENTED_EDGE('',*,*,#5879,.F.);
#8412=ORIENTED_EDGE('',*,*,#5880,.F.);
#8413=ORIENTED_EDGE('',*,*,#5881,.F.);
#8414=ORIENTED_EDGE('',*,*,#5882,.F.);
#8415=ORIENTED_EDGE('',*,*,#5883,.F.);
#8416=ORIENTED_EDGE('',*,*,#5884,.F.);
#8417=ORIENTED_EDGE('',*,*,#5885,.F.);
#8418=ORIENTED_EDGE('',*,*,#5877,.T.);
#8419=ORIENTED_EDGE('',*,*,#5886,.T.);
#8420=ORIENTED_EDGE('',*,*,#5884,.T.);
#8421=ORIENTED_EDGE('',*,*,#5887,.T.);
#8422=ORIENTED_EDGE('',*,*,#5803,.T.);
#8423=ORIENTED_EDGE('',*,*,#5888,.T.);
#8424=ORIENTED_EDGE('',*,*,#5885,.T.);
#8425=ORIENTED_EDGE('',*,*,#5889,.T.);
#8426=ORIENTED_EDGE('',*,*,#5890,.F.);
#8427=ORIENTED_EDGE('',*,*,#5891,.F.);
#8428=ORIENTED_EDGE('',*,*,#5892,.F.);
#8429=ORIENTED_EDGE('',*,*,#5891,.T.);
#8430=ORIENTED_EDGE('',*,*,#5893,.T.);
#8431=ORIENTED_EDGE('',*,*,#5881,.T.);
#8432=ORIENTED_EDGE('',*,*,#5894,.T.);
#8433=ORIENTED_EDGE('',*,*,#5883,.T.);
#8434=ORIENTED_EDGE('',*,*,#5895,.T.);
#8435=ORIENTED_EDGE('',*,*,#5892,.T.);
#8436=ORIENTED_EDGE('',*,*,#5896,.T.);
#8437=ORIENTED_EDGE('',*,*,#5801,.T.);
#8438=ORIENTED_EDGE('',*,*,#5897,.T.);
#8439=ORIENTED_EDGE('',*,*,#5890,.T.);
#8440=ORIENTED_EDGE('',*,*,#5898,.T.);
#8441=ORIENTED_EDGE('',*,*,#5799,.T.);
#8442=ORIENTED_EDGE('',*,*,#5899,.T.);
#8443=ORIENTED_EDGE('',*,*,#5882,.T.);
#8444=ORIENTED_EDGE('',*,*,#5900,.T.);
#8445=ORIENTED_EDGE('',*,*,#5880,.T.);
#8446=ORIENTED_EDGE('',*,*,#5901,.T.);
#8447=ORIENTED_EDGE('',*,*,#5878,.T.);
#8448=ORIENTED_EDGE('',*,*,#5902,.T.);
#8449=ORIENTED_EDGE('',*,*,#5797,.T.);
#8450=ORIENTED_EDGE('',*,*,#5903,.T.);
#8451=ORIENTED_EDGE('',*,*,#5879,.T.);
#8452=ORIENTED_EDGE('',*,*,#5904,.T.);
#8453=ORIENTED_EDGE('',*,*,#5898,.F.);
#8454=ORIENTED_EDGE('',*,*,#5895,.F.);
#8455=ORIENTED_EDGE('',*,*,#5888,.F.);
#8456=ORIENTED_EDGE('',*,*,#5802,.F.);
#8457=ORIENTED_EDGE('',*,*,#5720,.T.);
#8458=ORIENTED_EDGE('',*,*,#5804,.F.);
#8459=ORIENTED_EDGE('',*,*,#5889,.F.);
#8460=ORIENTED_EDGE('',*,*,#5886,.F.);
#8461=ORIENTED_EDGE('',*,*,#5903,.F.);
#8462=ORIENTED_EDGE('',*,*,#5796,.F.);
#8463=ORIENTED_EDGE('',*,*,#5736,.T.);
#8464=ORIENTED_EDGE('',*,*,#5749,.T.);
#8465=ORIENTED_EDGE('',*,*,#5894,.F.);
#8466=ORIENTED_EDGE('',*,*,#5902,.F.);
#8467=ORIENTED_EDGE('',*,*,#5887,.F.);
#8468=ORIENTED_EDGE('',*,*,#5896,.F.);
#8469=ORIENTED_EDGE('',*,*,#5666,.T.);
#8470=ORIENTED_EDGE('',*,*,#5682,.T.);
#8471=ORIENTED_EDGE('',*,*,#5679,.T.);
#8472=ORIENTED_EDGE('',*,*,#5676,.T.);
#8473=ORIENTED_EDGE('',*,*,#5673,.T.);
#8474=ORIENTED_EDGE('',*,*,#5670,.T.);
#8475=ORIENTED_EDGE('',*,*,#5685,.T.);
#8476=ORIENTED_EDGE('',*,*,#5701,.T.);
#8477=ORIENTED_EDGE('',*,*,#5698,.T.);
#8478=ORIENTED_EDGE('',*,*,#5695,.T.);
#8479=ORIENTED_EDGE('',*,*,#5692,.T.);
#8480=ORIENTED_EDGE('',*,*,#5689,.T.);
#8481=ORIENTED_EDGE('',*,*,#5712,.T.);
#8482=ORIENTED_EDGE('',*,*,#5709,.T.);
#8483=ORIENTED_EDGE('',*,*,#5706,.T.);
#8484=ORIENTED_EDGE('',*,*,#5704,.T.);
#8485=ORIENTED_EDGE('',*,*,#5899,.F.);
#8486=ORIENTED_EDGE('',*,*,#5798,.F.);
#8487=ORIENTED_EDGE('',*,*,#5904,.F.);
#8488=ORIENTED_EDGE('',*,*,#5901,.F.);
#8489=ORIENTED_EDGE('',*,*,#5897,.F.);
#8490=ORIENTED_EDGE('',*,*,#5800,.F.);
#8491=ORIENTED_EDGE('',*,*,#5900,.F.);
#8492=ORIENTED_EDGE('',*,*,#5893,.F.);
#9231=CYLINDRICAL_SURFACE('',#10372,0.25);
#9232=CYLINDRICAL_SURFACE('',#10374,0.25);
#9233=CYLINDRICAL_SURFACE('',#10376,0.25);
#9234=CYLINDRICAL_SURFACE('',#10378,0.25);
#9235=CYLINDRICAL_SURFACE('',#10400,0.15);
#9236=CYLINDRICAL_SURFACE('',#10402,0.15);
#9237=CYLINDRICAL_SURFACE('',#10405,0.15);
#9238=CYLINDRICAL_SURFACE('',#10408,0.15);
#9239=CYLINDRICAL_SURFACE('',#10410,0.17);
#9240=CYLINDRICAL_SURFACE('',#10412,0.17);
#9241=CYLINDRICAL_SURFACE('',#10436,0.4);
#9242=CYLINDRICAL_SURFACE('',#10437,0.4);
#9243=CYLINDRICAL_SURFACE('',#10460,0.1);
#9244=CYLINDRICAL_SURFACE('',#10464,0.1);
#9245=CYLINDRICAL_SURFACE('',#10478,0.3);
#9246=CYLINDRICAL_SURFACE('',#10483,0.3);
#9648=ADVANCED_FACE('',(#1622),#9231,.F.);
#9649=ADVANCED_FACE('',(#1623),#9232,.F.);
#9650=ADVANCED_FACE('',(#1624),#9233,.F.);
#9651=ADVANCED_FACE('',(#1625),#9234,.F.);
#9652=ADVANCED_FACE('',(#1626),#237,.T.);
#9653=ADVANCED_FACE('',(#1627),#238,.T.);
#9654=ADVANCED_FACE('',(#1628,#164,#165,#166),#1231,.F.);
#9655=ADVANCED_FACE('',(#1629),#1232,.F.);
#9656=ADVANCED_FACE('',(#1630),#1233,.F.);
#9657=ADVANCED_FACE('',(#1631),#1234,.F.);
#9658=ADVANCED_FACE('',(#1632),#1235,.F.);
#9659=ADVANCED_FACE('',(#1633),#1236,.F.);
#9660=ADVANCED_FACE('',(#1634),#1237,.F.);
#9661=ADVANCED_FACE('',(#1635,#167),#1238,.F.);
#9662=ADVANCED_FACE('',(#1636),#1239,.F.);
#9663=ADVANCED_FACE('',(#1637),#1240,.F.);
#9664=ADVANCED_FACE('',(#1638),#1241,.F.);
#9665=ADVANCED_FACE('',(#1639),#1242,.F.);
#9666=ADVANCED_FACE('',(#1640),#1243,.F.);
#9667=ADVANCED_FACE('',(#1641),#1244,.F.);
#9668=ADVANCED_FACE('',(#1642,#168),#1245,.F.);
#9669=ADVANCED_FACE('',(#1643),#9235,.F.);
#9670=ADVANCED_FACE('',(#1644),#9236,.F.);
#9671=ADVANCED_FACE('',(#1645),#9237,.F.);
#9672=ADVANCED_FACE('',(#1646),#9238,.F.);
#9673=ADVANCED_FACE('',(#1647),#9239,.F.);
#9674=ADVANCED_FACE('',(#1648),#9240,.F.);
#9675=ADVANCED_FACE('',(#1649),#1246,.F.);
#9676=ADVANCED_FACE('',(#1650),#1247,.F.);
#9677=ADVANCED_FACE('',(#1651),#1248,.F.);
#9678=ADVANCED_FACE('',(#1652),#1249,.F.);
#9679=ADVANCED_FACE('',(#1653),#1250,.F.);
#9680=ADVANCED_FACE('',(#1654),#1251,.F.);
#9681=ADVANCED_FACE('',(#1655),#1252,.F.);
#9682=ADVANCED_FACE('',(#1656,#169),#1253,.F.);
#9683=ADVANCED_FACE('',(#1657,#170),#1254,.F.);
#9684=ADVANCED_FACE('',(#1658),#1255,.F.);
#9685=ADVANCED_FACE('',(#1659),#1256,.F.);
#9686=ADVANCED_FACE('',(#1660),#1257,.F.);
#9687=ADVANCED_FACE('',(#1661),#1258,.F.);
#9688=ADVANCED_FACE('',(#1662),#1259,.F.);
#9689=ADVANCED_FACE('',(#1663),#1260,.T.);
#9690=ADVANCED_FACE('',(#1664),#1261,.T.);
#9691=ADVANCED_FACE('',(#1665),#1262,.T.);
#9692=ADVANCED_FACE('',(#1666),#1263,.T.);
#9693=ADVANCED_FACE('',(#1667),#1264,.T.);
#9694=ADVANCED_FACE('',(#1668,#171),#1265,.F.);
#9695=ADVANCED_FACE('',(#1669),#9241,.T.);
#9696=ADVANCED_FACE('',(#1670),#9242,.T.);
#9697=ADVANCED_FACE('',(#1671),#1266,.T.);
#9698=ADVANCED_FACE('',(#1672),#239,.T.);
#9699=ADVANCED_FACE('',(#1673),#240,.T.);
#9700=ADVANCED_FACE('',(#1674),#241,.T.);
#9701=ADVANCED_FACE('',(#1675),#242,.T.);
#9702=ADVANCED_FACE('',(#1676),#1267,.F.);
#9703=ADVANCED_FACE('',(#1677),#243,.T.);
#9704=ADVANCED_FACE('',(#1678),#244,.T.);
#9705=ADVANCED_FACE('',(#1679),#1268,.T.);
#9706=ADVANCED_FACE('',(#1680),#245,.T.);
#9707=ADVANCED_FACE('',(#1681),#246,.T.);
#9708=ADVANCED_FACE('',(#1682),#1269,.F.);
#9709=ADVANCED_FACE('',(#1683),#247,.T.);
#9710=ADVANCED_FACE('',(#1684),#248,.T.);
#9711=ADVANCED_FACE('',(#1685),#1270,.T.);
#9712=ADVANCED_FACE('',(#1686),#249,.T.);
#9713=ADVANCED_FACE('',(#1687),#250,.T.);
#9714=ADVANCED_FACE('',(#1688,#172,#173,#174),#1271,.F.);
#9715=ADVANCED_FACE('',(#1689),#251,.T.);
#9716=ADVANCED_FACE('',(#1690),#1272,.T.);
#9717=ADVANCED_FACE('',(#1691),#252,.T.);
#9718=ADVANCED_FACE('',(#1692),#253,.T.);
#9719=ADVANCED_FACE('',(#1693),#1273,.F.);
#9720=ADVANCED_FACE('',(#1694),#254,.T.);
#9721=ADVANCED_FACE('',(#1695),#255,.T.);
#9722=ADVANCED_FACE('',(#1696),#84,.F.);
#9723=ADVANCED_FACE('',(#1697),#85,.F.);
#9724=ADVANCED_FACE('',(#1698),#86,.F.);
#9725=ADVANCED_FACE('',(#1699),#9243,.F.);
#9726=ADVANCED_FACE('',(#1700),#256,.T.);
#9727=ADVANCED_FACE('',(#1701),#87,.F.);
#9728=ADVANCED_FACE('',(#1702),#9244,.F.);
#9729=ADVANCED_FACE('',(#1703),#257,.T.);
#9730=ADVANCED_FACE('',(#1704),#258,.T.);
#9731=ADVANCED_FACE('',(#1705),#259,.T.);
#9732=ADVANCED_FACE('',(#1706),#260,.T.);
#9733=ADVANCED_FACE('',(#1707),#1274,.T.);
#9734=ADVANCED_FACE('',(#1708),#88,.T.);
#9735=ADVANCED_FACE('',(#1709),#89,.T.);
#9736=ADVANCED_FACE('',(#1710),#90,.T.);
#9737=ADVANCED_FACE('',(#1711),#9245,.T.);
#9738=ADVANCED_FACE('',(#1712),#261,.F.);
#9739=ADVANCED_FACE('',(#1713),#91,.T.);
#9740=ADVANCED_FACE('',(#1714),#9246,.T.);
#9741=ADVANCED_FACE('',(#1715),#262,.F.);
#9742=ADVANCED_FACE('',(#1716),#263,.F.);
#9743=ADVANCED_FACE('',(#1717),#264,.F.);
#9744=ADVANCED_FACE('',(#1718),#265,.F.);
#9745=ADVANCED_FACE('',(#1719),#266,.F.);
#9746=ADVANCED_FACE('',(#1720),#267,.F.);
#9747=ADVANCED_FACE('',(#1721),#1275,.F.);
#9748=ADVANCED_FACE('',(#1722,#175,#176,#177,#178,#179,#180),#1276,.T.);
#9749=ADVANCED_FACE('',(#1723),#268,.F.);
#9750=ADVANCED_FACE('',(#1724),#1277,.F.);
#9894=CLOSED_SHELL('',(#9648,#9649,#9650,#9651,#9652,#9653,#9654,#9655,
#9656,#9657,#9658,#9659,#9660,#9661,#9662,#9663,#9664,#9665,#9666,#9667,
#9668,#9669,#9670,#9671,#9672,#9673,#9674,#9675,#9676,#9677,#9678,#9679,
#9680,#9681,#9682,#9683,#9684,#9685,#9686,#9687,#9688,#9689,#9690,#9691,
#9692,#9693,#9694,#9695,#9696,#9697,#9698,#9699,#9700,#9701,#9702,#9703,
#9704,#9705,#9706,#9707,#9708,#9709,#9710,#9711,#9712,#9713,#9714,#9715,
#9716,#9717,#9718,#9719,#9720,#9721,#9722,#9723,#9724,#9725,#9726,#9727,
#9728,#9729,#9730,#9731,#9732,#9733,#9734,#9735,#9736,#9737,#9738,#9739,
#9740,#9741,#9742,#9743,#9744,#9745,#9746,#9747,#9748,#9749,#9750));
#10371=AXIS2_PLACEMENT_3D('',#16983,#11737,#11738);
#10372=AXIS2_PLACEMENT_3D('',#16984,#11739,#11740);
#10373=AXIS2_PLACEMENT_3D('',#17011,#11741,#11742);
#10374=AXIS2_PLACEMENT_3D('',#17012,#11743,#11744);
#10375=AXIS2_PLACEMENT_3D('',#17035,#11745,#11746);
#10376=AXIS2_PLACEMENT_3D('',#17036,#11747,#11748);
#10377=AXIS2_PLACEMENT_3D('',#17059,#11749,#11750);
#10378=AXIS2_PLACEMENT_3D('',#17060,#11751,#11752);
#10379=AXIS2_PLACEMENT_3D('',#17087,#11753,#11754);
#10380=AXIS2_PLACEMENT_3D('',#17272,#11755,#11756);
#10381=AXIS2_PLACEMENT_3D('',#17286,#11759,#11760);
#10382=AXIS2_PLACEMENT_3D('',#17288,#11761,#11762);
#10383=AXIS2_PLACEMENT_3D('',#17290,#11763,#11764);
#10384=AXIS2_PLACEMENT_3D('',#17291,#11765,#11766);
#10385=AXIS2_PLACEMENT_3D('',#17300,#11771,#11772);
#10386=AXIS2_PLACEMENT_3D('',#17306,#11776,#11777);
#10387=AXIS2_PLACEMENT_3D('',#17312,#11781,#11782);
#10388=AXIS2_PLACEMENT_3D('',#17318,#11786,#11787);
#10389=AXIS2_PLACEMENT_3D('',#17324,#11791,#11792);
#10390=AXIS2_PLACEMENT_3D('',#17327,#11795,#11796);
#10391=AXIS2_PLACEMENT_3D('',#17329,#11797,#11798);
#10392=AXIS2_PLACEMENT_3D('',#17330,#11799,#11800);
#10393=AXIS2_PLACEMENT_3D('',#17339,#11805,#11806);
#10394=AXIS2_PLACEMENT_3D('',#17345,#11810,#11811);
#10395=AXIS2_PLACEMENT_3D('',#17351,#11815,#11816);
#10396=AXIS2_PLACEMENT_3D('',#17357,#11820,#11821);
#10397=AXIS2_PLACEMENT_3D('',#17363,#11825,#11826);
#10398=AXIS2_PLACEMENT_3D('',#17366,#11829,#11830);
#10399=AXIS2_PLACEMENT_3D('',#17368,#11831,#11832);
#10400=AXIS2_PLACEMENT_3D('',#17369,#11833,#11834);
#10401=AXIS2_PLACEMENT_3D('',#17371,#11835,#11836);
#10402=AXIS2_PLACEMENT_3D('',#17373,#11838,#11839);
#10403=AXIS2_PLACEMENT_3D('',#17375,#11840,#11841);
#10404=AXIS2_PLACEMENT_3D('',#17378,#11843,#11844);
#10405=AXIS2_PLACEMENT_3D('',#17379,#11845,#11846);
#10406=AXIS2_PLACEMENT_3D('',#17381,#11847,#11848);
#10407=AXIS2_PLACEMENT_3D('',#17384,#11850,#11851);
#10408=AXIS2_PLACEMENT_3D('',#17385,#11852,#11853);
#10409=AXIS2_PLACEMENT_3D('',#17387,#11854,#11855);
#10410=AXIS2_PLACEMENT_3D('',#17389,#11857,#11858);
#10411=AXIS2_PLACEMENT_3D('',#17392,#11860,#11861);
#10412=AXIS2_PLACEMENT_3D('',#17393,#11862,#11863);
#10413=AXIS2_PLACEMENT_3D('',#17396,#11865,#11866);
#10414=AXIS2_PLACEMENT_3D('',#17397,#11867,#11868);
#10415=AXIS2_PLACEMENT_3D('',#17406,#11873,#11874);
#10416=AXIS2_PLACEMENT_3D('',#17415,#11879,#11880);
#10417=AXIS2_PLACEMENT_3D('',#17424,#11885,#11886);
#10418=AXIS2_PLACEMENT_3D('',#17433,#11891,#11892);
#10419=AXIS2_PLACEMENT_3D('',#17442,#11897,#11898);
#10420=AXIS2_PLACEMENT_3D('',#17451,#11903,#11904);
#10421=AXIS2_PLACEMENT_3D('',#17460,#11909,#11910);
#10422=AXIS2_PLACEMENT_3D('',#17462,#11911,#11912);
#10423=AXIS2_PLACEMENT_3D('',#17463,#11913,#11914);
#10424=AXIS2_PLACEMENT_3D('',#17465,#11915,#11916);
#10425=AXIS2_PLACEMENT_3D('',#17466,#11917,#11918);
#10426=AXIS2_PLACEMENT_3D('',#17469,#11921,#11922);
#10427=AXIS2_PLACEMENT_3D('',#17472,#11925,#11926);
#10428=AXIS2_PLACEMENT_3D('',#17475,#11929,#11930);
#10429=AXIS2_PLACEMENT_3D('',#17481,#11934,#11935);
#10430=AXIS2_PLACEMENT_3D('',#17487,#11939,#11940);
#10431=AXIS2_PLACEMENT_3D('',#17532,#11942,#11943);
#10432=AXIS2_PLACEMENT_3D('',#17578,#11946,#11947);
#10433=AXIS2_PLACEMENT_3D('',#17656,#11951,#11952);
#10434=AXIS2_PLACEMENT_3D('',#17704,#11956,#11957);
#10435=AXIS2_PLACEMENT_3D('',#17720,#11961,#11962);
#10436=AXIS2_PLACEMENT_3D('',#18041,#11974,#11975);
#10437=AXIS2_PLACEMENT_3D('',#18043,#11977,#11978);
#10438=AXIS2_PLACEMENT_3D('',#18045,#11979,#11980);
#10439=AXIS2_PLACEMENT_3D('',#18047,#11982,#11983);
#10440=AXIS2_PLACEMENT_3D('',#18211,#11985,#11986);
#10441=AXIS2_PLACEMENT_3D('',#18212,#11987,#11988);
#10442=AXIS2_PLACEMENT_3D('',#18260,#11990,#11991);
#10443=AXIS2_PLACEMENT_3D('',#18378,#11993,#11994);
#10444=AXIS2_PLACEMENT_3D('',#18423,#11995,#11996);
#10445=AXIS2_PLACEMENT_3D('',#18515,#11998,#11999);
#10446=AXIS2_PLACEMENT_3D('',#18532,#12000,#12001);
#10447=AXIS2_PLACEMENT_3D('',#18652,#12003,#12004);
#10448=AXIS2_PLACEMENT_3D('',#18657,#12005,#12006);
#10449=AXIS2_PLACEMENT_3D('',#18709,#12008,#12009);
#10450=AXIS2_PLACEMENT_3D('',#18710,#12010,#12011);
#10451=AXIS2_PLACEMENT_3D('',#18711,#12012,#12013);
#10452=AXIS2_PLACEMENT_3D('',#18712,#12014,#12015);
#10453=AXIS2_PLACEMENT_3D('',#18713,#12016,#12017);
#10454=AXIS2_PLACEMENT_3D('',#18714,#12018,#12019);
#10455=AXIS2_PLACEMENT_3D('',#18716,#12020,#12021);
#10456=AXIS2_PLACEMENT_3D('',#18717,#12022,#12023);
#10457=AXIS2_PLACEMENT_3D('',#18718,#12024,#12025);
#10458=AXIS2_PLACEMENT_3D('',#18719,#12026,#12027);
#10459=AXIS2_PLACEMENT_3D('',#18720,#12028,#12029);
#10460=AXIS2_PLACEMENT_3D('',#18721,#12030,#12031);
#10461=AXIS2_PLACEMENT_3D('',#18742,#12032,#12033);
#10462=AXIS2_PLACEMENT_3D('',#18744,#12034,#12035);
#10463=AXIS2_PLACEMENT_3D('',#18745,#12036,#12037);
#10464=AXIS2_PLACEMENT_3D('',#18746,#12038,#12039);
#10465=AXIS2_PLACEMENT_3D('',#18836,#12041,#12042);
#10466=AXIS2_PLACEMENT_3D('',#18837,#12043,#12044);
#10467=AXIS2_PLACEMENT_3D('',#18840,#12045,#12046);
#10468=AXIS2_PLACEMENT_3D('',#18842,#12047,#12048);
#10469=AXIS2_PLACEMENT_3D('',#18843,#12049,#12050);
#10470=AXIS2_PLACEMENT_3D('',#18844,#12051,#12052);
#10471=AXIS2_PLACEMENT_3D('',#18847,#12053,#12054);
#10472=AXIS2_PLACEMENT_3D('',#18849,#12055,#12056);
#10473=AXIS2_PLACEMENT_3D('',#18850,#12057,#12058);
#10474=AXIS2_PLACEMENT_3D('',#18851,#12059,#12060);
#10475=AXIS2_PLACEMENT_3D('',#18854,#12061,#12062);
#10476=AXIS2_PLACEMENT_3D('',#18856,#12063,#12064);
#10477=AXIS2_PLACEMENT_3D('',#18857,#12065,#12066);
#10478=AXIS2_PLACEMENT_3D('',#18858,#12067,#12068);
#10479=AXIS2_PLACEMENT_3D('',#18889,#12071,#12072);
#10480=AXIS2_PLACEMENT_3D('',#18892,#12073,#12074);
#10481=AXIS2_PLACEMENT_3D('',#18894,#12075,#12076);
#10482=AXIS2_PLACEMENT_3D('',#18895,#12077,#12078);
#10483=AXIS2_PLACEMENT_3D('',#18896,#12079,#12080);
#10484=AXIS2_PLACEMENT_3D('',#19069,#12083,#12084);
#10485=AXIS2_PLACEMENT_3D('',#19070,#12085,#12086);
#10486=AXIS2_PLACEMENT_3D('',#19087,#12087,#12088);
#11737=DIRECTION('axis',(0.,0.,1.));
#11738=DIRECTION('refdir',(1.,0.,0.));
#11739=DIRECTION('center_axis',(0.,0.,-1.));
#11740=DIRECTION('ref_axis',(1.,0.,0.));
#11741=DIRECTION('center_axis',(0.,0.,1.));
#11742=DIRECTION('ref_axis',(1.,0.,0.));
#11743=DIRECTION('center_axis',(0.,0.,-1.));
#11744=DIRECTION('ref_axis',(1.,0.,0.));
#11745=DIRECTION('center_axis',(0.,0.,1.));
#11746=DIRECTION('ref_axis',(1.,0.,0.));
#11747=DIRECTION('center_axis',(0.,0.,-1.));
#11748=DIRECTION('ref_axis',(1.,0.,0.));
#11749=DIRECTION('center_axis',(0.,0.,1.));
#11750=DIRECTION('ref_axis',(1.,0.,0.));
#11751=DIRECTION('center_axis',(0.,0.,-1.));
#11752=DIRECTION('ref_axis',(1.,0.,0.));
#11753=DIRECTION('center_axis',(0.,0.,1.));
#11754=DIRECTION('ref_axis',(1.,0.,0.));
#11755=DIRECTION('center_axis',(4.10828654779316E-33,-1.13946463231163E-19,
1.));
#11756=DIRECTION('ref_axis',(1.,0.,-4.10828654779316E-33));
#11757=DIRECTION('',(0.,1.,1.13946463231163E-19));
#11758=DIRECTION('',(0.,-1.,-1.13946463231163E-19));
#11759=DIRECTION('center_axis',(4.10828654779316E-33,-1.13946463231163E-19,
1.));
#11760=DIRECTION('ref_axis',(1.,0.,0.));
#11761=DIRECTION('center_axis',(4.10828654779316E-33,-1.13946463231163E-19,
1.));
#11762=DIRECTION('ref_axis',(1.,0.,0.));
#11763=DIRECTION('center_axis',(4.10828654779316E-33,-1.13946463231163E-19,
1.));
#11764=DIRECTION('ref_axis',(1.,0.,0.));
#11765=DIRECTION('center_axis',(0.86602540378444,0.499999999999998,0.));
#11766=DIRECTION('ref_axis',(0.499999999999998,-0.86602540378444,0.));
#11767=DIRECTION('',(0.499999999999998,-0.86602540378444,-9.86805318295791E-20));
#11768=DIRECTION('',(0.,0.,-1.));
#11769=DIRECTION('',(0.499999999999998,-0.86602540378444,0.));
#11770=DIRECTION('',(0.,0.,-1.));
#11771=DIRECTION('center_axis',(1.60246890531964E-16,1.,0.));
#11772=DIRECTION('ref_axis',(1.,-1.60246890531964E-16,0.));
#11773=DIRECTION('',(1.,-1.60246890531964E-16,-4.12654611421307E-33));
#11774=DIRECTION('',(0.,0.,-1.));
#11775=DIRECTION('',(1.,-1.60246890531964E-16,0.));
#11776=DIRECTION('center_axis',(-0.86602540378444,0.499999999999998,0.));
#11777=DIRECTION('ref_axis',(0.499999999999998,0.86602540378444,0.));
#11778=DIRECTION('',(0.499999999999998,0.86602540378444,9.86805318295749E-20));
#11779=DIRECTION('',(0.,0.,-1.));
#11780=DIRECTION('',(0.499999999999998,0.86602540378444,0.));
#11781=DIRECTION('center_axis',(-0.86602540378444,-0.499999999999998,0.));
#11782=DIRECTION('ref_axis',(-0.499999999999998,0.86602540378444,0.));
#11783=DIRECTION('',(-0.499999999999998,0.86602540378444,9.86805318295791E-20));
#11784=DIRECTION('',(0.,0.,-1.));
#11785=DIRECTION('',(-0.499999999999998,0.86602540378444,0.));
#11786=DIRECTION('center_axis',(-1.60246890531964E-16,-1.,0.));
#11787=DIRECTION('ref_axis',(-1.,1.60246890531964E-16,0.));
#11788=DIRECTION('',(-1.,1.60246890531964E-16,4.12654611421307E-33));
#11789=DIRECTION('',(0.,0.,-1.));
#11790=DIRECTION('',(-1.,1.60246890531964E-16,0.));
#11791=DIRECTION('center_axis',(0.86602540378444,-0.499999999999998,0.));
#11792=DIRECTION('ref_axis',(-0.499999999999998,-0.86602540378444,0.));
#11793=DIRECTION('',(-0.499999999999998,-0.86602540378444,-9.86805318295749E-20));
#11794=DIRECTION('',(-0.499999999999998,-0.86602540378444,0.));
#11795=DIRECTION('center_axis',(0.,0.,-1.));
#11796=DIRECTION('ref_axis',(-1.,0.,0.));
#11797=DIRECTION('center_axis',(0.,0.,1.));
#11798=DIRECTION('ref_axis',(1.,0.,0.));
#11799=DIRECTION('center_axis',(0.866025403784439,0.5,0.));
#11800=DIRECTION('ref_axis',(0.5,-0.866025403784439,0.));
#11801=DIRECTION('',(0.5,-0.866025403784439,-9.86805318295789E-20));
#11802=DIRECTION('',(0.,0.,-1.));
#11803=DIRECTION('',(0.5,-0.866025403784439,0.));
#11804=DIRECTION('',(0.,0.,-1.));
#11805=DIRECTION('center_axis',(1.60246890531964E-16,1.,0.));
#11806=DIRECTION('ref_axis',(1.,-1.60246890531964E-16,0.));
#11807=DIRECTION('',(1.,-1.60246890531964E-16,-4.12654611421307E-33));
#11808=DIRECTION('',(0.,0.,-1.));
#11809=DIRECTION('',(1.,-1.60246890531964E-16,0.));
#11810=DIRECTION('center_axis',(-0.866025403784438,0.5,0.));
#11811=DIRECTION('ref_axis',(0.5,0.866025403784438,0.));
#11812=DIRECTION('',(0.5,0.866025403784438,9.86805318295748E-20));
#11813=DIRECTION('',(0.,0.,-1.));
#11814=DIRECTION('',(0.5,0.866025403784438,0.));
#11815=DIRECTION('center_axis',(-0.866025403784439,-0.499999999999999,0.));
#11816=DIRECTION('ref_axis',(-0.499999999999999,0.866025403784439,0.));
#11817=DIRECTION('',(-0.499999999999999,0.866025403784439,9.8680531829579E-20));
#11818=DIRECTION('',(0.,0.,-1.));
#11819=DIRECTION('',(-0.499999999999999,0.866025403784439,0.));
#11820=DIRECTION('center_axis',(-1.60246890531964E-16,-1.,0.));
#11821=DIRECTION('ref_axis',(-1.,1.60246890531964E-16,0.));
#11822=DIRECTION('',(-1.,1.60246890531964E-16,4.12654611421307E-33));
#11823=DIRECTION('',(0.,0.,-1.));
#11824=DIRECTION('',(-1.,1.60246890531964E-16,0.));
#11825=DIRECTION('center_axis',(0.866025403784439,-0.5,0.));
#11826=DIRECTION('ref_axis',(-0.5,-0.866025403784439,0.));
#11827=DIRECTION('',(-0.5,-0.866025403784439,-9.86805318295748E-20));
#11828=DIRECTION('',(-0.5,-0.866025403784439,0.));
#11829=DIRECTION('center_axis',(0.,0.,-1.));
#11830=DIRECTION('ref_axis',(-1.,0.,0.));
#11831=DIRECTION('center_axis',(0.,0.,1.));
#11832=DIRECTION('ref_axis',(1.,0.,0.));
#11833=DIRECTION('center_axis',(0.,0.,-1.));
#11834=DIRECTION('ref_axis',(1.,0.,0.));
#11835=DIRECTION('center_axis',(-4.10828654779316E-33,1.13946463231163E-19,
-1.));
#11836=DIRECTION('ref_axis',(1.,0.,0.));
#11837=DIRECTION('',(0.,0.,-1.));
#11838=DIRECTION('center_axis',(0.,0.,-1.));
#11839=DIRECTION('ref_axis',(1.,0.,0.));
#11840=DIRECTION('center_axis',(-4.10828654779316E-33,1.13946463231163E-19,
-1.));
#11841=DIRECTION('ref_axis',(1.,0.,0.));
#11842=DIRECTION('',(0.,0.,-1.));
#11843=DIRECTION('center_axis',(4.10828654779316E-33,-1.13946463231163E-19,
1.));
#11844=DIRECTION('ref_axis',(1.,0.,0.));
#11845=DIRECTION('center_axis',(0.,0.,-1.));
#11846=DIRECTION('ref_axis',(1.,0.,0.));
#11847=DIRECTION('center_axis',(-4.10828654779316E-33,1.13946463231163E-19,
-1.));
#11848=DIRECTION('ref_axis',(1.,0.,0.));
#11849=DIRECTION('',(0.,0.,-1.));
#11850=DIRECTION('center_axis',(4.10828654779316E-33,-1.13946463231163E-19,
1.));
#11851=DIRECTION('ref_axis',(1.,0.,0.));
#11852=DIRECTION('center_axis',(0.,0.,-1.));
#11853=DIRECTION('ref_axis',(1.,0.,0.));
#11854=DIRECTION('center_axis',(-4.10828654779316E-33,1.13946463231163E-19,
-1.));
#11855=DIRECTION('ref_axis',(1.,0.,0.));
#11856=DIRECTION('',(0.,0.,-1.));
#11857=DIRECTION('center_axis',(0.,0.,-1.));
#11858=DIRECTION('ref_axis',(1.,0.,0.));
#11859=DIRECTION('',(0.,0.,-1.));
#11860=DIRECTION('center_axis',(0.,0.,1.));
#11861=DIRECTION('ref_axis',(1.,0.,0.));
#11862=DIRECTION('center_axis',(0.,0.,-1.));
#11863=DIRECTION('ref_axis',(1.,0.,0.));
#11864=DIRECTION('',(0.,0.,-1.));
#11865=DIRECTION('center_axis',(0.,0.,1.));
#11866=DIRECTION('ref_axis',(1.,0.,0.));
#11867=DIRECTION('center_axis',(0.,-1.,0.));
#11868=DIRECTION('ref_axis',(-1.,0.,0.));
#11869=DIRECTION('',(0.0523359562429438,0.,0.998629534754574));
#11870=DIRECTION('',(1.,0.,0.));
#11871=DIRECTION('',(-0.0523359562429438,0.,-0.998629534754574));
#11872=DIRECTION('',(1.,0.,0.));
#11873=DIRECTION('center_axis',(0.,-1.,0.));
#11874=DIRECTION('ref_axis',(-1.,0.,0.));
#11875=DIRECTION('',(0.,0.,-1.));
#11876=DIRECTION('',(1.,0.,0.));
#11877=DIRECTION('',(0.,0.,1.));
#11878=DIRECTION('',(1.,0.,0.));
#11879=DIRECTION('center_axis',(0.,-1.,0.));
#11880=DIRECTION('ref_axis',(-1.,0.,0.));
#11881=DIRECTION('',(0.,0.,-1.));
#11882=DIRECTION('',(1.,0.,0.));
#11883=DIRECTION('',(0.,0.,1.));
#11884=DIRECTION('',(1.,0.,0.));
#11885=DIRECTION('center_axis',(0.,-1.,0.));
#11886=DIRECTION('ref_axis',(-1.,0.,0.));
#11887=DIRECTION('',(0.,0.,-1.));
#11888=DIRECTION('',(1.,0.,0.));
#11889=DIRECTION('',(0.,0.,1.));
#11890=DIRECTION('',(1.,0.,0.));
#11891=DIRECTION('center_axis',(0.,1.,0.));
#11892=DIRECTION('ref_axis',(1.,0.,0.));
#11893=DIRECTION('',(-0.0523359562429438,0.,-0.998629534754574));
#11894=DIRECTION('',(-1.,0.,0.));
#11895=DIRECTION('',(0.0523359562429438,0.,0.998629534754574));
#11896=DIRECTION('',(-1.,0.,0.));
#11897=DIRECTION('center_axis',(0.,1.,0.));
#11898=DIRECTION('ref_axis',(1.,0.,0.));
#11899=DIRECTION('',(0.,0.,1.));
#11900=DIRECTION('',(-1.,0.,0.));
#11901=DIRECTION('',(0.,0.,-1.));
#11902=DIRECTION('',(-1.,0.,0.));
#11903=DIRECTION('center_axis',(0.,1.,0.));
#11904=DIRECTION('ref_axis',(1.,0.,0.));
#11905=DIRECTION('',(0.,0.,1.));
#11906=DIRECTION('',(-1.,0.,0.));
#11907=DIRECTION('',(0.,0.,-1.));
#11908=DIRECTION('',(-1.,0.,0.));
#11909=DIRECTION('center_axis',(0.,0.,1.));
#11910=DIRECTION('ref_axis',(1.,0.,0.));
#11911=DIRECTION('center_axis',(0.,0.,1.));
#11912=DIRECTION('ref_axis',(1.,0.,0.));
#11913=DIRECTION('center_axis',(0.,0.,1.));
#11914=DIRECTION('ref_axis',(1.,0.,0.));
#11915=DIRECTION('center_axis',(0.,0.,1.));
#11916=DIRECTION('ref_axis',(1.,0.,0.));
#11917=DIRECTION('center_axis',(0.,0.,1.));
#11918=DIRECTION('ref_axis',(1.,0.,0.));
#11919=DIRECTION('',(0.,1.,0.));
#11920=DIRECTION('',(0.,-1.,0.));
#11921=DIRECTION('center_axis',(0.,0.,1.));
#11922=DIRECTION('ref_axis',(1.,0.,0.));
#11923=DIRECTION('',(0.,-1.,0.));
#11924=DIRECTION('',(0.,1.,0.));
#11925=DIRECTION('center_axis',(0.,0.,1.));
#11926=DIRECTION('ref_axis',(1.,0.,0.));
#11927=DIRECTION('',(0.,-1.,0.));
#11928=DIRECTION('',(0.,1.,0.));
#11929=DIRECTION('center_axis',(0.,0.,1.));
#11930=DIRECTION('ref_axis',(1.,0.,0.));
#11931=DIRECTION('',(0.,-1.,0.));
#11932=DIRECTION('',(-1.,0.,0.));
#11933=DIRECTION('',(0.,1.,0.));
#11934=DIRECTION('center_axis',(0.,1.,0.));
#11935=DIRECTION('ref_axis',(1.,0.,0.));
#11936=DIRECTION('',(0.,0.,1.));
#11937=DIRECTION('',(-1.,0.,0.));
#11938=DIRECTION('',(0.,0.,-1.));
#11939=DIRECTION('center_axis',(-1.,0.,0.));
#11940=DIRECTION('ref_axis',(0.,-1.,0.));
#11941=DIRECTION('',(0.,-1.,0.));
#11942=DIRECTION('center_axis',(1.,0.,0.));
#11943=DIRECTION('ref_axis',(0.,1.,0.));
#11944=DIRECTION('',(0.,1.,0.));
#11945=DIRECTION('',(0.,1.,0.));
#11946=DIRECTION('center_axis',(1.,0.,0.));
#11947=DIRECTION('ref_axis',(0.,1.,0.));
#11948=DIRECTION('',(0.,1.,0.));
#11949=DIRECTION('',(0.,1.,1.13946463231163E-19));
#11950=DIRECTION('',(0.,1.,0.));
#11951=DIRECTION('center_axis',(1.,0.,0.));
#11952=DIRECTION('ref_axis',(0.,1.,0.));
#11953=DIRECTION('',(0.,1.,0.));
#11954=DIRECTION('',(0.,1.,1.13946463231163E-19));
#11955=DIRECTION('',(0.,1.,0.));
#11956=DIRECTION('center_axis',(0.998629534754574,0.,-0.0523359562429438));
#11957=DIRECTION('ref_axis',(-0.0523359562429438,0.,-0.998629534754574));
#11958=DIRECTION('',(0.,-1.,0.));
#11959=DIRECTION('',(-5.97168109510197E-21,-1.,-1.13946463231163E-19));
#11960=DIRECTION('',(0.,-1.,0.));
#11961=DIRECTION('center_axis',(0.,0.,1.));
#11962=DIRECTION('ref_axis',(1.,0.,0.));
#11963=DIRECTION('',(0.,-1.,0.));
#11964=DIRECTION('',(0.,-1.,0.));
#11965=DIRECTION('',(0.,-1.,0.));
#11966=DIRECTION('',(0.,1.,0.));
#11967=DIRECTION('',(0.,-1.,0.));
#11968=DIRECTION('',(0.,1.,0.));
#11969=DIRECTION('',(0.,-1.,0.));
#11970=DIRECTION('',(0.,-1.,0.));
#11971=DIRECTION('',(0.,-1.,0.));
#11972=DIRECTION('',(0.,1.,0.));
#11973=DIRECTION('',(0.,1.,0.));
#11974=DIRECTION('center_axis',(0.,0.,1.));
#11975=DIRECTION('ref_axis',(1.,0.,0.));
#11976=DIRECTION('',(0.,0.,-1.));
#11977=DIRECTION('center_axis',(0.,0.,1.));
#11978=DIRECTION('ref_axis',(1.,0.,0.));
#11979=DIRECTION('center_axis',(4.10828654779316E-33,-1.13946463231163E-19,
1.));
#11980=DIRECTION('ref_axis',(1.,0.,0.));
#11981=DIRECTION('',(0.,0.,-1.));
#11982=DIRECTION('center_axis',(1.,0.,0.));
#11983=DIRECTION('ref_axis',(0.,1.,0.));
#11984=DIRECTION('',(0.,1.,1.13946463231163E-19));
#11985=DIRECTION('center_axis',(0.99852593895705,0.0542765992849681,9.38276897523041E-9));
#11986=DIRECTION('ref_axis',(0.0541946171271057,-0.99701772369063,0.0549418066794405));
#11987=DIRECTION('center_axis',(4.10828654779316E-33,-1.13946463231163E-19,
1.));
#11988=DIRECTION('ref_axis',(1.,0.,-4.10828654779316E-33));
#11989=DIRECTION('',(5.97168109510217E-21,-1.,-1.13946463231163E-19));
#11990=DIRECTION('center_axis',(-1.,0.,0.));
#11991=DIRECTION('ref_axis',(0.,-1.,0.));
#11992=DIRECTION('',(0.,-1.,-1.13946463231163E-19));
#11993=DIRECTION('center_axis',(4.10828654779316E-33,-1.13946463231163E-19,
1.));
#11994=DIRECTION('ref_axis',(1.,0.,-4.10828654779316E-33));
#11995=DIRECTION('center_axis',(-1.,0.,0.));
#11996=DIRECTION('ref_axis',(0.,-1.,0.));
#11997=DIRECTION('',(0.,-1.,-1.13946463231163E-19));
#11998=DIRECTION('center_axis',(4.10828654779316E-33,-1.13946463231163E-19,
1.));
#11999=DIRECTION('ref_axis',(1.,0.,-4.10828654779316E-33));
#12000=DIRECTION('center_axis',(-1.,0.,0.));
#12001=DIRECTION('ref_axis',(0.,-1.,0.));
#12002=DIRECTION('',(0.,-1.,-1.13946463231163E-19));
#12003=DIRECTION('center_axis',(-0.996961060527779,0.0779015005717205,0.));
#12004=DIRECTION('ref_axis',(0.,0.,1.));
#12005=DIRECTION('center_axis',(4.10828654779316E-33,-1.13946463231163E-19,
1.));
#12006=DIRECTION('ref_axis',(1.,0.,-4.10828654779316E-33));
#12007=DIRECTION('',(5.97168109510197E-21,1.,1.13946463231163E-19));
#12008=DIRECTION('center_axis',(-0.996961060527779,-0.0779015005717276,
-4.485055189269E-15));
#12009=DIRECTION('ref_axis',(-0.0777791112471086,0.995394757055134,0.0560329142626144));
#12010=DIRECTION('center_axis',(-0.377317868652411,-0.840644185582845,0.388521015186253));
#12011=DIRECTION('ref_axis',(-0.58566693710526,0.541587807512093,0.603056287203763));
#12012=DIRECTION('center_axis',(7.41164423166535E-16,1.,0.));
#12013=DIRECTION('ref_axis',(0.,0.,1.));
#12014=DIRECTION('center_axis',(0.0522650005536027,-0.0520548592672972,
0.997275619547472));
#12015=DIRECTION('ref_axis',(-0.998629534754574,7.40148683083438E-16,0.0523359562429445));
#12016=DIRECTION('center_axis',(0.376559988603802,-0.837471124372148,0.396036224133039));
#12017=DIRECTION('ref_axis',(0.577069986161316,0.546481578685729,0.606916893181374));
#12018=DIRECTION('center_axis',(0.998525938475037,-0.0542766081525538,0.));
#12019=DIRECTION('ref_axis',(0.,0.,1.));
#12020=DIRECTION('center_axis',(-0.0522648366634829,-0.0521149007022807,
0.997272492337641));
#12021=DIRECTION('ref_axis',(0.0541946171271058,0.99701772369063,0.0549418066794413));
#12022=DIRECTION('center_axis',(5.32220538281047E-11,1.,-1.01553728389566E-9));
#12023=DIRECTION('ref_axis',(0.998629534754574,0.,0.0523359562429456));
#12024=DIRECTION('center_axis',(0.37731786865241,-0.840644185582843,-0.388521015186259));
#12025=DIRECTION('ref_axis',(-0.585666937105255,-0.541587807512096,0.603056287203765));
#12026=DIRECTION('center_axis',(0.0522650005536027,0.0520548592672965,0.997275619547472));
#12027=DIRECTION('ref_axis',(-0.0777791112471059,-0.995394757055134,0.0560329142626137));
#12028=DIRECTION('center_axis',(0.,-1.,0.));
#12029=DIRECTION('ref_axis',(-0.998629534754574,0.,0.0523359562429439));
#12030=DIRECTION('center_axis',(5.97168109510197E-21,1.,1.13946463231163E-19));
#12031=DIRECTION('ref_axis',(-0.688354575693753,0.,0.725374371012288));
#12032=DIRECTION('center_axis',(-0.376559987018669,-0.837471124206646,-0.396036225990193));
#12033=DIRECTION('ref_axis',(0.577069983350267,-0.54648157893936,0.606916895625808));
#12034=DIRECTION('center_axis',(-0.0522648366634817,0.0521149007022785,
0.997272492337641));
#12035=DIRECTION('ref_axis',(0.998629534754574,0.,0.052335956242946));
#12036=DIRECTION('center_axis',(1.01693095242295E-9,-1.,0.));
#12037=DIRECTION('ref_axis',(0.,0.,1.));
#12038=DIRECTION('center_axis',(5.97168109510217E-21,-1.,-1.13946463231163E-19));
#12039=DIRECTION('ref_axis',(0.688354575693753,0.,0.725374371012289));
#12040=DIRECTION('',(-5.97168109510217E-21,1.,1.13946463231163E-19));
#12041=DIRECTION('center_axis',(-0.998629534754574,0.,-0.0523359562429455));
#12042=DIRECTION('ref_axis',(-0.0523359562429455,0.,0.998629534754574));
#12043=DIRECTION('center_axis',(-0.377317868652411,-0.840644185582845,0.388521015186254));
#12044=DIRECTION('ref_axis',(-0.585666937105261,0.541587807512092,0.603056287203763));
#12045=DIRECTION('center_axis',(7.41164423166535E-16,1.,0.));
#12046=DIRECTION('ref_axis',(0.,0.,1.));
#12047=DIRECTION('center_axis',(-0.996961060527779,-0.0779015005717276,
-4.485055189269E-15));
#12048=DIRECTION('ref_axis',(-0.0777791112471086,0.995394757055134,0.0560329142626144));
#12049=DIRECTION('center_axis',(0.0522650005536027,-0.0520548592672972,
0.997275619547472));
#12050=DIRECTION('ref_axis',(-0.998629534754574,7.40148683083438E-16,0.0523359562429445));
#12051=DIRECTION('center_axis',(0.376559988603802,-0.837471124372148,0.396036224133039));
#12052=DIRECTION('ref_axis',(0.577069986161311,0.546481578685732,0.606916893181376));
#12053=DIRECTION('center_axis',(0.998525938475037,-0.0542766081525538,0.));
#12054=DIRECTION('ref_axis',(0.,0.,1.));
#12055=DIRECTION('center_axis',(5.32220538281047E-11,1.,-1.01553728389566E-9));
#12056=DIRECTION('ref_axis',(0.998629534754574,0.,0.0523359562429456));
#12057=DIRECTION('center_axis',(-0.0522648366634829,-0.0521149007022807,
0.997272492337641));
#12058=DIRECTION('ref_axis',(0.0541946171271058,0.99701772369063,0.0549418066794413));
#12059=DIRECTION('center_axis',(0.37731786865241,-0.840644185582843,-0.388521015186259));
#12060=DIRECTION('ref_axis',(-0.585666937105255,-0.541587807512095,0.603056287203766));
#12061=DIRECTION('center_axis',(-0.996961060527779,0.0779015005717205,0.));
#12062=DIRECTION('ref_axis',(0.,0.,1.));
#12063=DIRECTION('center_axis',(0.,-1.,0.));
#12064=DIRECTION('ref_axis',(-0.998629534754574,0.,0.0523359562429439));
#12065=DIRECTION('center_axis',(0.0522650005536027,0.0520548592672965,0.997275619547472));
#12066=DIRECTION('ref_axis',(-0.0777791112471059,-0.995394757055134,0.0560329142626137));
#12067=DIRECTION('center_axis',(5.97168109510197E-21,1.,1.13946463231163E-19));
#12068=DIRECTION('ref_axis',(-0.688354575693753,0.,0.725374371012289));
#12069=DIRECTION('',(-5.97168109510197E-21,-1.,-1.13946463231163E-19));
#12070=DIRECTION('',(5.97168109510197E-21,1.,1.13946463231163E-19));
#12071=DIRECTION('center_axis',(-0.376559987018669,-0.837471124206646,-0.396036225990194));
#12072=DIRECTION('ref_axis',(0.577069983350267,-0.546481578939359,0.606916895625808));
#12073=DIRECTION('center_axis',(-0.0522648366634817,0.0521149007022785,
0.997272492337641));
#12074=DIRECTION('ref_axis',(0.998629534754574,0.,0.052335956242946));
#12075=DIRECTION('center_axis',(1.01693095242295E-9,-1.,0.));
#12076=DIRECTION('ref_axis',(0.,0.,1.));
#12077=DIRECTION('center_axis',(0.99852593895705,0.0542765992849681,9.38276897523041E-9));
#12078=DIRECTION('ref_axis',(0.0541946171271057,-0.99701772369063,0.0549418066794405));
#12079=DIRECTION('center_axis',(5.97168109510217E-21,-1.,-1.13946463231163E-19));
#12080=DIRECTION('ref_axis',(0.688354575693753,0.,0.725374371012289));
#12081=DIRECTION('',(-5.97168109510217E-21,1.,1.13946463231163E-19));
#12082=DIRECTION('',(5.97168109510217E-21,-1.,-1.13946463231163E-19));
#12083=DIRECTION('center_axis',(0.998629534754574,0.,-0.0523359562429438));
#12084=DIRECTION('ref_axis',(-0.0523359562429438,0.,-0.998629534754574));
#12085=DIRECTION('center_axis',(4.10828654779316E-33,-1.13946463231163E-19,
1.));
#12086=DIRECTION('ref_axis',(1.,0.,-4.10828654779316E-33));
#12087=DIRECTION('center_axis',(-0.998629534754574,0.,-0.0523359562429455));
#12088=DIRECTION('ref_axis',(-0.0523359562429455,0.,0.998629534754574));
#16983=CARTESIAN_POINT('',(0.,0.,0.));
#16984=CARTESIAN_POINT('Origin',(8.1,-1.,0.7));
#16985=CARTESIAN_POINT('',(7.94916965151797,-1.19937453693185,0.7));
#16986=CARTESIAN_POINT('',(8.26514540988519,-1.18768855477586,0.7));
#16987=CARTESIAN_POINT('Ctrl Pts',(7.94916965151797,-1.19937453693185,0.7));
#16988=CARTESIAN_POINT('Ctrl Pts',(7.97160858810976,-1.21634998764782,0.7));
#16989=CARTESIAN_POINT('Ctrl Pts',(7.99739856866269,-1.22989011121344,0.69528529300377));
#16990=CARTESIAN_POINT('Ctrl Pts',(8.03944443766207,-1.24298414277179,0.688517705185315));
#16991=CARTESIAN_POINT('Ctrl Pts',(8.05362924383607,-1.24609346022897,0.686388676887586));
#16992=CARTESIAN_POINT('Ctrl Pts',(8.075506183533,-1.24890990228851,0.684139035126277));
#16993=CARTESIAN_POINT('Ctrl Pts',(8.08297567221474,-1.24953307703463,0.683546226354886));
#16994=CARTESIAN_POINT('Ctrl Pts',(8.0940066533036,-1.24995288972095,0.68299521602547));
#16995=CARTESIAN_POINT('Ctrl Pts',(8.09752287926269,-1.25001251279495,0.68286729538075));
#16996=CARTESIAN_POINT('Ctrl Pts',(8.10293413375911,-1.249989933108,0.682747340264197));
#16997=CARTESIAN_POINT('Ctrl Pts',(8.10482478940148,-1.24996059450444,0.682719828470948));
#16998=CARTESIAN_POINT('Ctrl Pts',(8.10828546792054,-1.24986760009171,0.682696100760705));
#16999=CARTESIAN_POINT('Ctrl Pts',(8.10985478687837,-1.24981062779486,0.682695370268813));
#17000=CARTESIAN_POINT('Ctrl Pts',(8.11326464342549,-1.24965465239671,0.682715595753076));
#17001=CARTESIAN_POINT('Ctrl Pts',(8.11510409202247,-1.2495501177419,0.682740330911594));
#17002=CARTESIAN_POINT('Ctrl Pts',(8.12014207260669,-1.24920790966494,0.682845651127781));
#17003=CARTESIAN_POINT('Ctrl Pts',(8.12333423895876,-1.24892926854386,0.682953992816581));
#17004=CARTESIAN_POINT('Ctrl Pts',(8.139194120874,-1.2472372768871,0.683691668462565));
#17005=CARTESIAN_POINT('Ctrl Pts',(8.15164141295685,-1.2449338270761,0.684918799511701));
#17006=CARTESIAN_POINT('Ctrl Pts',(8.19196937649467,-1.23428099896052,0.690212518998986));
#17007=CARTESIAN_POINT('Ctrl Pts',(8.21811504697062,-1.22213176592155,0.695755006185672));
#17008=CARTESIAN_POINT('Ctrl Pts',(8.24962874265135,-1.20052913769617,0.699397421419897));
#17009=CARTESIAN_POINT('Ctrl Pts',(8.25758631484639,-1.19433973204149,0.7));
#17010=CARTESIAN_POINT('Ctrl Pts',(8.26514540988519,-1.18768855477586,0.7));
#17011=CARTESIAN_POINT('Origin',(8.1,-1.,0.7));
#17012=CARTESIAN_POINT('Origin',(2.7,1.,0.7));
#17013=CARTESIAN_POINT('',(2.8076286513348,1.22564590451442,0.7));
#17014=CARTESIAN_POINT('',(2.57739843082973,1.21787348447435,0.7));
#17015=CARTESIAN_POINT('Ctrl Pts',(2.80762864495888,1.22564590575571,0.7));
#17016=CARTESIAN_POINT('Ctrl Pts',(2.78743249310418,1.23527907171202,0.7));
#17017=CARTESIAN_POINT('Ctrl Pts',(2.76507271635938,1.24261561512899,0.698430289974852));
#17018=CARTESIAN_POINT('Ctrl Pts',(2.73219941643314,1.24807722603274,0.696876198609429));
#17019=CARTESIAN_POINT('Ctrl Pts',(2.72335305886828,1.24906618730719,0.696525251810408));
#17020=CARTESIAN_POINT('Ctrl Pts',(2.71018695034311,1.24982905432238,0.696188910804419));
#17021=CARTESIAN_POINT('Ctrl Pts',(2.70590779780308,1.24996687586326,0.696107915309552));
#17022=CARTESIAN_POINT('Ctrl Pts',(2.69921702211412,1.25001037316246,0.696030339680738));
#17023=CARTESIAN_POINT('Ctrl Pts',(2.69680890442544,1.24999123464332,0.696012302673685));
#17024=CARTESIAN_POINT('Ctrl Pts',(2.69234597975348,1.24989125947742,0.695997601992606));
#17025=CARTESIAN_POINT('Ctrl Pts',(2.69029169500035,1.24981988388707,0.69599819279703));
#17026=CARTESIAN_POINT('Ctrl Pts',(2.6857660481318,1.24960673159635,0.696015705561832));
#17027=CARTESIAN_POINT('Ctrl Pts',(2.68329599580702,1.24945360531346,0.696035938105249));
#17028=CARTESIAN_POINT('Ctrl Pts',(2.67625328071593,1.24891193026541,0.696123377063474));
#17029=CARTESIAN_POINT('Ctrl Pts',(2.67169109188753,1.24843439216159,0.696216059649547));
#17030=CARTESIAN_POINT('Ctrl Pts',(2.64765560351845,1.24524789167778,0.696873729305584));
#17031=CARTESIAN_POINT('Ctrl Pts',(2.62857598726268,1.24037162800668,0.698048768812303));
#17032=CARTESIAN_POINT('Ctrl Pts',(2.59902076831046,1.22902239593109,0.699541037747764));
#17033=CARTESIAN_POINT('Ctrl Pts',(2.58799157881597,1.22383445108162,0.7));
#17034=CARTESIAN_POINT('Ctrl Pts',(2.57739843082979,1.21787348447436,0.7));
#17035=CARTESIAN_POINT('Origin',(2.7,1.,0.7));
#17036=CARTESIAN_POINT('Origin',(2.7,-1.,0.7));
#17037=CARTESIAN_POINT('',(2.57739843082979,-1.21787348447436,0.7));
#17038=CARTESIAN_POINT('',(2.80762864495888,-1.22564590575571,0.7));
#17039=CARTESIAN_POINT('Ctrl Pts',(2.57739843082979,-1.21787348447436,0.7));
#17040=CARTESIAN_POINT('Ctrl Pts',(2.59689796709118,-1.22884624579732,0.7));
#17041=CARTESIAN_POINT('Ctrl Pts',(2.61871070177046,-1.23767364961455,0.698430520021629));
#17042=CARTESIAN_POINT('Ctrl Pts',(2.6511387549791,-1.24533993869645,0.696876447160353));
#17043=CARTESIAN_POINT('Ctrl Pts',(2.65989793055836,-1.24692336726652,0.696525471319567));
#17044=CARTESIAN_POINT('Ctrl Pts',(2.67298219502323,-1.24857266139659,0.696189053183015));
#17045=CARTESIAN_POINT('Ctrl Pts',(2.67724223626036,-1.24899884484677,0.696108027479433));
#17046=CARTESIAN_POINT('Ctrl Pts',(2.68391475503581,-1.24949361628703,0.696030400846995));
#17047=CARTESIAN_POINT('Ctrl Pts',(2.68631866330158,-1.24963697932539,0.69601234479389));
#17048=CARTESIAN_POINT('Ctrl Pts',(2.69077815115796,-1.24983831390468,0.695997608323079));
#17049=CARTESIAN_POINT('Ctrl Pts',(2.69283257145917,-1.24990568929416,0.695998182544699));
#17050=CARTESIAN_POINT('Ctrl Pts',(2.69736230434386,-1.24999833696454,0.696015659042177));
#17051=CARTESIAN_POINT('Ctrl Pts',(2.69983707579759,-1.25001219669429,0.696035872086962));
#17052=CARTESIAN_POINT('Ctrl Pts',(2.70690037992806,-1.24994687665095,0.696123257636812));
#17053=CARTESIAN_POINT('Ctrl Pts',(2.71148446565418,-1.24977820005943,0.696215908504701));
#17054=CARTESIAN_POINT('Ctrl Pts',(2.73568105999059,-1.24822038288304,0.696873447340259));
#17055=CARTESIAN_POINT('Ctrl Pts',(2.75504695022812,-1.24464213141243,0.698048515307351));
#17056=CARTESIAN_POINT('Ctrl Pts',(2.78530198112344,-1.2353118289445,0.699540950501024));
#17057=CARTESIAN_POINT('Ctrl Pts',(2.79665680001786,-1.23087925931356,0.7));
#17058=CARTESIAN_POINT('Ctrl Pts',(2.80762864495888,-1.22564590575571,0.7));
#17059=CARTESIAN_POINT('Origin',(2.7,-1.,0.7));
#17060=CARTESIAN_POINT('Origin',(8.1,1.,0.7));
#17061=CARTESIAN_POINT('',(8.26514540988519,1.18768855477586,0.7));
#17062=CARTESIAN_POINT('',(7.94916965249954,1.19937453719419,0.7));
#17063=CARTESIAN_POINT('Ctrl Pts',(8.26514540988519,1.18768855477586,0.7));
#17064=CARTESIAN_POINT('Ctrl Pts',(8.24402114884725,1.20627559516199,0.7));
#17065=CARTESIAN_POINT('Ctrl Pts',(8.21930102059268,1.22168408824046,0.695284768760077));
#17066=CARTESIAN_POINT('Ctrl Pts',(8.17833936508797,1.23784683595578,0.688517484674842));
#17067=CARTESIAN_POINT('Ctrl Pts',(8.16442627443898,1.24199461640617,0.686388979601913));
#17068=CARTESIAN_POINT('Ctrl Pts',(8.14282164862934,1.24641910835203,0.684139556285851));
#17069=CARTESIAN_POINT('Ctrl Pts',(8.13541969045672,1.24759243465272,0.683546718614312));
#17070=CARTESIAN_POINT('Ctrl Pts',(8.12445132655127,1.24882623938238,0.682995554842566));
#17071=CARTESIAN_POINT('Ctrl Pts',(8.12094947916695,1.24914555886372,0.68286756899844));
#17072=CARTESIAN_POINT('Ctrl Pts',(8.11555178799172,1.24952297970176,0.682747494033431));
#17073=CARTESIAN_POINT('Ctrl Pts',(8.11366421100955,1.24963346420394,0.682719937279798));
#17074=CARTESIAN_POINT('Ctrl Pts',(8.11020620287515,1.24979651712922,0.682696124556263));
#17075=CARTESIAN_POINT('Ctrl Pts',(8.10863696767328,1.24985569708818,0.682695355189016));
#17076=CARTESIAN_POINT('Ctrl Pts',(8.10522484403353,1.249952190393,0.682715496638402));
#17077=CARTESIAN_POINT('Ctrl Pts',(8.10338263267786,1.24998390529834,0.682740187713169));
#17078=CARTESIAN_POINT('Ctrl Pts',(8.09833277498968,1.25001501472208,0.682845394223802));
#17079=CARTESIAN_POINT('Ctrl Pts',(8.09512844909059,1.24997307323179,0.682953673497893));
#17080=CARTESIAN_POINT('Ctrl Pts',(8.07918314804204,1.24945780552822,0.683691186949858));
#17081=CARTESIAN_POINT('Ctrl Pts',(8.06659630270856,1.24808001426183,0.684918585227095));
#17082=CARTESIAN_POINT('Ctrl Pts',(8.02558960427868,1.24043495378573,0.69021260546313));
#17083=CARTESIAN_POINT('Ctrl Pts',(7.9986188553413,1.2302509517108,0.695754623970086));
#17084=CARTESIAN_POINT('Ctrl Pts',(7.96559475436581,1.21103543221342,0.69939729083119));
#17085=CARTESIAN_POINT('Ctrl Pts',(7.95720051358587,1.20545002552208,0.7));
#17086=CARTESIAN_POINT('Ctrl Pts',(7.94916965151797,1.19937453693185,0.7));
#17087=CARTESIAN_POINT('Origin',(8.1,1.,0.7));
#17088=CARTESIAN_POINT('Ctrl Pts',(1.1,1.14549341399196,0.7));
#17089=CARTESIAN_POINT('Ctrl Pts',(1.89984199608574,1.1957170361627,0.7));
#17090=CARTESIAN_POINT('Ctrl Pts',(2.70080437300401,1.2273695200909,0.7));
#17091=CARTESIAN_POINT('Ctrl Pts',(3.50204003610941,1.24374118183538,0.7));
#17092=CARTESIAN_POINT('Ctrl Pts',(1.09819048660397,1.17431102498992,0.7));
#17093=CARTESIAN_POINT('Ctrl Pts',(1.89847848223077,1.22458382597074,0.70000077422621));
#17094=CARTESIAN_POINT('Ctrl Pts',(2.69984520196781,1.25626413437997,0.699999727319846));
#17095=CARTESIAN_POINT('Ctrl Pts',(3.50144932661635,1.27265074030048,0.700000000000001));
#17096=CARTESIAN_POINT('Ctrl Pts',(1.09505363188407,1.22426736091617,0.676703190608825));
#17097=CARTESIAN_POINT('Ctrl Pts',(1.89610976425884,1.27462253270773,0.67666760713801));
#17098=CARTESIAN_POINT('Ctrl Pts',(2.69818680938115,1.3063522351595,0.67664530655333));
#17099=CARTESIAN_POINT('Ctrl Pts',(3.50042536655637,1.322763754511,0.676632802377821));
#17100=CARTESIAN_POINT('Ctrl Pts',(1.09381704710221,1.24396073223232,0.627109609335854));
#17101=CARTESIAN_POINT('Ctrl Pts',(1.89518106151152,1.29430885982199,0.62701751976321));
#17102=CARTESIAN_POINT('Ctrl Pts',(2.69753328610131,1.32603127467068,0.626959208652505));
#17103=CARTESIAN_POINT('Ctrl Pts',(3.50002334924346,1.34243864233338,0.626926882269943));
#17104=CARTESIAN_POINT('Ctrl Pts',(1.09374258853658,1.24514653057163,0.605486452199395));
#17105=CARTESIAN_POINT('Ctrl Pts',(1.89512529323683,1.29547288309274,0.605377720397184));
#17106=CARTESIAN_POINT('Ctrl Pts',(2.69749615303001,1.32718177535833,0.605308474776761));
#17107=CARTESIAN_POINT('Ctrl Pts',(3.5,1.34358136363184,0.605270327458635));
#17108=CARTESIAN_POINT('',(1.1,1.14549341399195,0.7));
#17109=CARTESIAN_POINT('Ctrl Pts',(1.1,1.14549341399196,0.7));
#17110=CARTESIAN_POINT('Ctrl Pts',(1.59210562457523,1.17639367564078,0.7));
#17111=CARTESIAN_POINT('Ctrl Pts',(2.08463535466703,1.20026407570248,0.7));
#17112=CARTESIAN_POINT('Ctrl Pts',(2.57739190516306,1.2178709162388,0.7));
#17113=CARTESIAN_POINT('',(1.1,1.24553911298206,0.605485603995113));
#17114=CARTESIAN_POINT('Ctrl Pts',(1.1,1.14549341399196,0.7));
#17115=CARTESIAN_POINT('Ctrl Pts',(1.1,1.15341616150799,0.7));
#17116=CARTESIAN_POINT('Ctrl Pts',(1.1000012416168,1.16127613060545,0.699006361583129));
#17117=CARTESIAN_POINT('Ctrl Pts',(1.10000231308998,1.16893252943985,0.697119293189023));
#17118=CARTESIAN_POINT('Ctrl Pts',(1.10000291357081,1.17322337016277,0.696061732044743));
#17119=CARTESIAN_POINT('Ctrl Pts',(1.10000345673767,1.17745032641463,0.694722535963768));
#17120=CARTESIAN_POINT('Ctrl Pts',(1.10000379529503,1.18158693416151,0.693112479763539));
#17121=CARTESIAN_POINT('Ctrl Pts',(1.1000044034764,1.18901789868739,0.690220189452084));
#17122=CARTESIAN_POINT('Ctrl Pts',(1.1000042334852,1.19607766167095,0.686488065947256));
#17123=CARTESIAN_POINT('Ctrl Pts',(1.10000339376692,1.2026196529327,0.681996646156542));
#17124=CARTESIAN_POINT('Ctrl Pts',(1.10000293249552,1.20621327895058,0.67952943359521));
#17125=CARTESIAN_POINT('Ctrl Pts',(1.10000228571683,1.20965039763183,0.676832226278619));
#17126=CARTESIAN_POINT('Ctrl Pts',(1.10000171524363,1.21290279159005,0.673912896410569));
#17127=CARTESIAN_POINT('Ctrl Pts',(1.10000115816795,1.2160788033717,0.671062126739188));
#17128=CARTESIAN_POINT('Ctrl Pts',(1.10000066850715,1.2190594221245,0.668016750164662));
#17129=CARTESIAN_POINT('Ctrl Pts',(1.10000067525152,1.22182202639256,0.664788091882127));
#17130=CARTESIAN_POINT('Ctrl Pts',(1.10000068775799,1.22694487635592,0.658801012170571));
#17131=CARTESIAN_POINT('Ctrl Pts',(1.10000222199399,1.23132099043293,0.652185071179834));
#17132=CARTESIAN_POINT('Ctrl Pts',(1.10000276904041,1.23488987417606,0.64510534613808));
#17133=CARTESIAN_POINT('Ctrl Pts',(1.10000282439334,1.23525099193115,0.644388983656765));
#17134=CARTESIAN_POINT('Ctrl Pts',(1.10000287212626,1.23560380546488,0.64366785367332));
#17135=CARTESIAN_POINT('Ctrl Pts',(1.10000291138002,1.23594822450451,0.642942116631622));
#17136=CARTESIAN_POINT('Ctrl Pts',(1.10000329911404,1.23935026814133,0.635773555081239));
#17137=CARTESIAN_POINT('Ctrl Pts',(1.10000258010782,1.24189771450306,0.628240464257889));
#17138=CARTESIAN_POINT('Ctrl Pts',(1.10000149084855,1.24353681278199,0.620511076118615));
#17139=CARTESIAN_POINT('Ctrl Pts',(1.10000079446814,1.24458471384188,0.615569557890241));
#17140=CARTESIAN_POINT('Ctrl Pts',(1.10000000111128,1.24526049271905,0.610547146027233));
#17141=CARTESIAN_POINT('Ctrl Pts',(1.09999999916631,1.24553911263843,0.605485603997432));
#17142=CARTESIAN_POINT('',(3.5,1.34358136363184,0.605270327458635));
#17143=CARTESIAN_POINT('Ctrl Pts',(3.5,1.34358136363184,0.605270327458635));
#17144=CARTESIAN_POINT('Ctrl Pts',(2.6995848679345,1.32722445934619,0.605308375488923));
#17145=CARTESIAN_POINT('Ctrl Pts',(1.89930203168261,1.29563783986497,0.605377360150118));
#17146=CARTESIAN_POINT('Ctrl Pts',(1.09999999916631,1.24553911263843,0.605485603997431));
#17147=CARTESIAN_POINT('',(3.5,1.24369946473792,0.7));
#17148=CARTESIAN_POINT('Ctrl Pts',(3.5,1.34358136363184,0.605270327458635));
#17149=CARTESIAN_POINT('Ctrl Pts',(3.5,1.34316359984937,0.613184373088104));
#17150=CARTESIAN_POINT('Ctrl Pts',(3.50000057901142,1.34177887744868,0.621008021569537));
#17151=CARTESIAN_POINT('Ctrl Pts',(3.50000082863025,1.33951086762262,0.628580534231506));
#17152=CARTESIAN_POINT('Ctrl Pts',(3.50000096811,1.33824356956914,0.632811834486987));
#17153=CARTESIAN_POINT('Ctrl Pts',(3.50000102536574,1.33669948631919,0.636964759527324));
#17154=CARTESIAN_POINT('Ctrl Pts',(3.50000098105742,1.334886463945,0.641009258704104));
#17155=CARTESIAN_POINT('Ctrl Pts',(3.50000090179773,1.3316432906201,0.648244145614236));
#17156=CARTESIAN_POINT('Ctrl Pts',(3.50000044940971,1.3275777080273,0.655054131048541));
#17157=CARTESIAN_POINT('Ctrl Pts',(3.50000027423476,1.32275302640998,0.661275670751788));
#17158=CARTESIAN_POINT('Ctrl Pts',(3.50000024156065,1.32185311357394,0.66243612938574));
#17159=CARTESIAN_POINT('Ctrl Pts',(3.50000022115524,1.32092666334894,0.663576045687695));
#17160=CARTESIAN_POINT('Ctrl Pts',(3.50000022069074,1.31997391848392,0.664694242102532));
#17161=CARTESIAN_POINT('Ctrl Pts',(3.50000021976176,1.31806844339147,0.666930617752677));
#17162=CARTESIAN_POINT('Ctrl Pts',(3.50000029790302,1.31605782519,0.669080165434128));
#17163=CARTESIAN_POINT('Ctrl Pts',(3.50000040488465,1.31394946763378,0.671139079687271));
#17164=CARTESIAN_POINT('Ctrl Pts',(3.50000069329649,1.3082655455861,0.6766897075128));
#17165=CARTESIAN_POINT('Ctrl Pts',(3.5000011432336,1.30193818666762,0.681521899278667));
#17166=CARTESIAN_POINT('Ctrl Pts',(3.50000129797765,1.29513115062548,0.68558123547136));
#17167=CARTESIAN_POINT('Ctrl Pts',(3.50000139624096,1.2908086457691,0.688158936000333));
#17168=CARTESIAN_POINT('Ctrl Pts',(3.50000139493488,1.28629176508013,0.690424313967808));
#17169=CARTESIAN_POINT('Ctrl Pts',(3.50000129141552,1.28161680488022,0.692354162840695));
#17170=CARTESIAN_POINT('Ctrl Pts',(3.50000112941005,1.27430059661786,0.695374333209024));
#17171=CARTESIAN_POINT('Ctrl Pts',(3.5000007162179,1.26668229982361,0.697540280949125));
#17172=CARTESIAN_POINT('Ctrl Pts',(3.50000038344698,1.25890895215876,0.698782355543395));
#17173=CARTESIAN_POINT('Ctrl Pts',(3.50000016866387,1.25389173534334,0.699584038140014));
#17174=CARTESIAN_POINT('Ctrl Pts',(3.4999999993056,1.24880933504677,0.69999999987784));
#17175=CARTESIAN_POINT('Ctrl Pts',(3.49999999991873,1.24369946470729,0.7));
#17176=CARTESIAN_POINT('Ctrl Pts',(2.80762377174497,1.22564400643366,0.7));
#17177=CARTESIAN_POINT('Ctrl Pts',(3.03837960601223,1.23298334400942,0.7));
#17178=CARTESIAN_POINT('Ctrl Pts',(3.26917843294065,1.23897560812206,0.7));
#17179=CARTESIAN_POINT('Ctrl Pts',(3.49999999991873,1.24369946470729,0.7));
#17180=CARTESIAN_POINT('Ctrl Pts',(7.29709043526678,1.22049830417059,0.7));
#17181=CARTESIAN_POINT('Ctrl Pts',(8.19846709497879,1.19422430779862,0.7));
#17182=CARTESIAN_POINT('Ctrl Pts',(9.09944331332256,1.15544418981837,0.7));
#17183=CARTESIAN_POINT('Ctrl Pts',(10.,1.10900986674273,0.7));
#17184=CARTESIAN_POINT('Ctrl Pts',(7.29793284700474,1.24939875264889,0.7));
#17185=CARTESIAN_POINT('Ctrl Pts',(8.19957769811722,1.22310890030201,0.699999704549177));
#17186=CARTESIAN_POINT('Ctrl Pts',(9.10076698492607,1.18430758604571,0.700000491839571));
#17187=CARTESIAN_POINT('Ctrl Pts',(10.0014871213396,1.13785139984992,0.7));
#17188=CARTESIAN_POINT('Ctrl Pts',(7.29939288958794,1.29948813715084,0.676630595533454));
#17189=CARTESIAN_POINT('Ctrl Pts',(8.20149954052228,1.27317186922949,0.676644146017132));
#17190=CARTESIAN_POINT('Ctrl Pts',(9.10306300621911,1.23433322993607,0.676664155483857));
#17191=CARTESIAN_POINT('Ctrl Pts',(10.0040646682326,1.18784086746588,0.676686753673613));
#17192=CARTESIAN_POINT('Ctrl Pts',(7.29996660609513,1.31917051289423,0.626939603849942));
#17193=CARTESIAN_POINT('Ctrl Pts',(8.20225661204673,1.29285896783792,0.626974637782525));
#17194=CARTESIAN_POINT('Ctrl Pts',(9.10396596140606,1.25402923300358,0.627026849623412));
#17195=CARTESIAN_POINT('Ctrl Pts',(10.0050807923581,1.20754778500352,0.627085325222079));
#17196=CARTESIAN_POINT('Ctrl Pts',(7.29999999953093,1.32031613471704,0.605285370449856));
#17197=CARTESIAN_POINT('Ctrl Pts',(8.20230020786565,1.29401302889245,0.605326714446839));
#17198=CARTESIAN_POINT('Ctrl Pts',(9.10401978846669,1.25519559703033,0.605388684776982));
#17199=CARTESIAN_POINT('Ctrl Pts',(10.0051416645797,1.20872835322339,0.605457722909465));
#17200=CARTESIAN_POINT('',(7.29999999989017,1.22041345054104,0.7));
#17201=CARTESIAN_POINT('Ctrl Pts',(7.29999999978094,1.22041345055303,0.7));
#17202=CARTESIAN_POINT('Ctrl Pts',(7.51641201913776,1.21409884615949,0.7));
#17203=CARTESIAN_POINT('Ctrl Pts',(7.73280095443524,1.20706364503479,0.7));
#17204=CARTESIAN_POINT('Ctrl Pts',(7.94916654146952,1.19937499621344,0.7));
#17205=CARTESIAN_POINT('',(7.29999999953133,1.3203161347307,0.605285370449834));
#17206=CARTESIAN_POINT('Ctrl Pts',(7.29999999989087,1.22041345054982,0.7));
#17207=CARTESIAN_POINT('Ctrl Pts',(7.30000000079355,1.22832360919786,0.699999999740221));
#17208=CARTESIAN_POINT('Ctrl Pts',(7.29999941101664,1.23617007614594,0.699006006469939));
#17209=CARTESIAN_POINT('Ctrl Pts',(7.29999889581476,1.24381267896118,0.697118889344366));
#17210=CARTESIAN_POINT('Ctrl Pts',(7.29999860583198,1.24811433880851,0.696056720321257));
#17211=CARTESIAN_POINT('Ctrl Pts',(7.29999834128398,1.25235147078274,0.694710570513598));
#17212=CARTESIAN_POINT('Ctrl Pts',(7.29999817264931,1.25649739217805,0.693091458416622));
#17213=CARTESIAN_POINT('Ctrl Pts',(7.29999787070862,1.26392067210813,0.690192435210923));
#17214=CARTESIAN_POINT('Ctrl Pts',(7.29999793286912,1.27097116792553,0.686452948287278));
#17215=CARTESIAN_POINT('Ctrl Pts',(7.2999983123982,1.27750284616821,0.681954753865011));
#17216=CARTESIAN_POINT('Ctrl Pts',(7.2999985213788,1.28109939299731,0.679477906983553));
#17217=CARTESIAN_POINT('Ctrl Pts',(7.29999881895966,1.28453837241868,0.676770138671336));
#17218=CARTESIAN_POINT('Ctrl Pts',(7.29999908362886,1.28779148632494,0.673839551409954));
#17219=CARTESIAN_POINT('Ctrl Pts',(7.29999934163235,1.29096267037196,0.670982771155867));
#17220=CARTESIAN_POINT('Ctrl Pts',(7.29999957112158,1.2939379836903,0.667931525418885));
#17221=CARTESIAN_POINT('Ctrl Pts',(7.29999957127586,1.29669488996436,0.664697318929259));
#17222=CARTESIAN_POINT('Ctrl Pts',(7.29999957156178,1.30180432468448,0.658703293276094));
#17223=CARTESIAN_POINT('Ctrl Pts',(7.29999886995656,1.30616650855536,0.652082235935803));
#17224=CARTESIAN_POINT('Ctrl Pts',(7.29999863193158,1.30972187224872,0.644999691185358));
#17225=CARTESIAN_POINT('Ctrl Pts',(7.29999860759325,1.31008541227461,0.644275492840527));
#17226=CARTESIAN_POINT('Ctrl Pts',(7.29999858692673,1.31044047656777,0.643546449710686));
#17227=CARTESIAN_POINT('Ctrl Pts',(7.29999857034625,1.31078697300061,0.642812727646596));
#17228=CARTESIAN_POINT('Ctrl Pts',(7.29999840819729,1.31417553742296,0.635637287305567));
#17229=CARTESIAN_POINT('Ctrl Pts',(7.29999876577208,1.31670951795567,0.628098908385918));
#17230=CARTESIAN_POINT('Ctrl Pts',(7.29999928780719,1.3183355664444,0.620365998324013));
#17231=CARTESIAN_POINT('Ctrl Pts',(7.29999962266353,1.3193785856694,0.615405768714856));
#17232=CARTESIAN_POINT('Ctrl Pts',(7.3,1.32004717656055,0.610364828659741));
#17233=CARTESIAN_POINT('Ctrl Pts',(7.3,1.32031613470337,0.605285370449877));
#17234=CARTESIAN_POINT('',(10.,1.20899340483173,0.605457329065657));
#17235=CARTESIAN_POINT('Ctrl Pts',(9.99999999968202,1.20899340489109,0.605457329065633));
#17236=CARTESIAN_POINT('Ctrl Pts',(9.10058974048747,1.25534320916473,0.605388449123016));
#17237=CARTESIAN_POINT('Ctrl Pts',(8.20058408060299,1.29406305600824,0.605326635812744));
#17238=CARTESIAN_POINT('Ctrl Pts',(7.29999999953093,1.32031613471704,0.605285370449856));
#17239=CARTESIAN_POINT('',(9.99999999523418,1.1090098672342,0.7));
#17240=CARTESIAN_POINT('Ctrl Pts',(9.99999999968202,1.20899340489109,0.605457329065633));
#17241=CARTESIAN_POINT('Ctrl Pts',(9.99999999887489,1.20856043137698,0.613368813757176));
#17242=CARTESIAN_POINT('Ctrl Pts',(9.99999852309337,1.20715974444566,0.621187403383205));
#17243=CARTESIAN_POINT('Ctrl Pts',(9.99999786661901,1.20487567413208,0.628752957409046));
#17244=CARTESIAN_POINT('Ctrl Pts',(9.9999975031266,1.20361097553651,0.63294203403));
#17245=CARTESIAN_POINT('Ctrl Pts',(9.99999733971606,1.20207445367248,0.63705356322819));
#17246=CARTESIAN_POINT('Ctrl Pts',(9.99999742766416,1.20027388348257,0.64105842070465));
#17247=CARTESIAN_POINT('Ctrl Pts',(9.9999975865154,1.19702170610966,0.6482919664668));
#17248=CARTESIAN_POINT('Ctrl Pts',(9.99999868569093,1.19294650045069,0.655099368158521));
#17249=CARTESIAN_POINT('Ctrl Pts',(9.9999991134218,1.18811276085989,0.661317774786376));
#17250=CARTESIAN_POINT('Ctrl Pts',(9.99999919410111,1.18720101282252,0.662490701033652));
#17251=CARTESIAN_POINT('Ctrl Pts',(9.99999924414009,1.18626214680169,0.663642601192937));
#17252=CARTESIAN_POINT('Ctrl Pts',(9.99999924372355,1.18529642131707,0.664772262763739));
#17253=CARTESIAN_POINT('Ctrl Pts',(9.99999924291654,1.18342543943696,0.666960851926287));
#17254=CARTESIAN_POINT('Ctrl Pts',(9.99999905429896,1.18145367213587,0.669066014649603));
#17255=CARTESIAN_POINT('Ctrl Pts',(9.99999879621773,1.17938809187152,0.671084194359814));
#17256=CARTESIAN_POINT('Ctrl Pts',(9.99999808597787,1.17370361260899,0.676638227242868));
#17257=CARTESIAN_POINT('Ctrl Pts',(9.9999969699445,1.16737553754052,0.681473799108647));
#17258=CARTESIAN_POINT('Ctrl Pts',(9.99999660204079,1.16056788011185,0.685537070165577));
#17259=CARTESIAN_POINT('Ctrl Pts',(9.99999636768906,1.15623145667386,0.688125341392612));
#17260=CARTESIAN_POINT('Ctrl Pts',(9.99999638726733,1.15169947441128,0.690399565850749));
#17261=CARTESIAN_POINT('Ctrl Pts',(9.99999666360534,1.14700857532255,0.692336497939236));
#17262=CARTESIAN_POINT('Ctrl Pts',(9.99999709503399,1.13968497812548,0.695360504669253));
#17263=CARTESIAN_POINT('Ctrl Pts',(9.99999815490668,1.13205884654683,0.697530003145419));
#17264=CARTESIAN_POINT('Ctrl Pts',(9.99999900983214,1.12427739544825,0.698775573347137));
#17265=CARTESIAN_POINT('Ctrl Pts',(9.99999956314479,1.11924119569193,0.699581713521624));
#17266=CARTESIAN_POINT('Ctrl Pts',(10.,1.11413933950174,0.7));
#17267=CARTESIAN_POINT('Ctrl Pts',(10.,1.10900986674273,0.7));
#17268=CARTESIAN_POINT('Ctrl Pts',(8.26514054272776,1.18768929227839,0.7));
#17269=CARTESIAN_POINT('Ctrl Pts',(8.84359655063997,1.16547286645366,0.7));
#17270=CARTESIAN_POINT('Ctrl Pts',(9.42188471826001,1.13881853081542,0.7));
#17271=CARTESIAN_POINT('Ctrl Pts',(9.99999999522154,1.10900986698912,0.7));
#17272=CARTESIAN_POINT('Origin',(5.4,-8.11656130105013E-18,0.7));
#17273=CARTESIAN_POINT('',(7.3,-1.22041345053557,0.7));
#17274=CARTESIAN_POINT('Ctrl Pts',(7.94916654049851,-1.19937499624794,0.7));
#17275=CARTESIAN_POINT('Ctrl Pts',(7.73280095382446,-1.20706364505454,0.7));
#17276=CARTESIAN_POINT('Ctrl Pts',(7.51641201888728,-1.21409884616656,0.7));
#17277=CARTESIAN_POINT('Ctrl Pts',(7.29999999989085,-1.22041345054982,0.7));
#17278=CARTESIAN_POINT('',(7.3,-0.712777777777778,0.7));
#17279=CARTESIAN_POINT('',(10.,-1.10900986674244,0.7));
#17280=CARTESIAN_POINT('',(10.,0.653773457742722,0.7));
#17281=CARTESIAN_POINT('Ctrl Pts',(10.,-1.10900986674273,0.7));
#17282=CARTESIAN_POINT('Ctrl Pts',(9.42188472144661,-1.13881853066854,0.7));
#17283=CARTESIAN_POINT('Ctrl Pts',(8.84359655223373,-1.16547286639245,0.7));
#17284=CARTESIAN_POINT('Ctrl Pts',(8.26514054272776,-1.18768929227839,0.7));
#17285=CARTESIAN_POINT('',(7.95,-1.,0.7));
#17286=CARTESIAN_POINT('Origin',(8.1,-1.,0.7));
#17287=CARTESIAN_POINT('',(7.95,1.,0.7));
#17288=CARTESIAN_POINT('Origin',(8.1,1.,0.7));
#17289=CARTESIAN_POINT('',(8.4,-4.89858719658942E-17,0.7));
#17290=CARTESIAN_POINT('Origin',(8.8,0.,0.7));
#17291=CARTESIAN_POINT('Origin',(8.97320508075689,0.3,0.9));
#17292=CARTESIAN_POINT('',(8.97320508075689,0.3,0.9));
#17293=CARTESIAN_POINT('',(9.14641016151377,0.,0.9));
#17294=CARTESIAN_POINT('',(8.59150635094611,0.961121593216771,0.9));
#17295=CARTESIAN_POINT('',(8.97320508075689,0.3,0.6));
#17296=CARTESIAN_POINT('',(8.97320508075689,0.3,0.9));
#17297=CARTESIAN_POINT('',(9.14641016151377,0.,0.6));
#17298=CARTESIAN_POINT('',(9.14641016151377,0.,0.6));
#17299=CARTESIAN_POINT('',(9.14641016151377,0.,0.9));
#17300=CARTESIAN_POINT('Origin',(8.62679491924311,0.3,0.9));
#17301=CARTESIAN_POINT('',(8.62679491924311,0.3,0.9));
#17302=CARTESIAN_POINT('',(7.01339745962156,0.3,0.9));
#17303=CARTESIAN_POINT('',(8.62679491924311,0.3,0.6));
#17304=CARTESIAN_POINT('',(8.62679491924311,0.3,0.9));
#17305=CARTESIAN_POINT('',(8.97320508075689,0.3,0.6));
#17306=CARTESIAN_POINT('Origin',(8.45358983848623,5.55111512312578E-17,
0.9));
#17307=CARTESIAN_POINT('',(8.45358983848623,4.24230095489963E-17,0.9));
#17308=CARTESIAN_POINT('',(8.07189110867545,-0.661121593216771,0.9));
#17309=CARTESIAN_POINT('',(8.45358983848623,5.55111512312578E-17,0.6));
#17310=CARTESIAN_POINT('',(8.45358983848623,4.24230095489963E-17,0.9));
#17311=CARTESIAN_POINT('',(8.62679491924311,0.3,0.6));
#17312=CARTESIAN_POINT('Origin',(8.62679491924311,-0.3,0.9));
#17313=CARTESIAN_POINT('',(8.62679491924311,-0.3,0.9));
#17314=CARTESIAN_POINT('',(8.15849364905389,0.511121593216771,0.9));
#17315=CARTESIAN_POINT('',(8.62679491924311,-0.3,0.6));
#17316=CARTESIAN_POINT('',(8.62679491924311,-0.3,0.9));
#17317=CARTESIAN_POINT('',(8.45358983848623,4.24230095489963E-17,0.6));
#17318=CARTESIAN_POINT('Origin',(8.97320508075689,-0.3,0.9));
#17319=CARTESIAN_POINT('',(8.97320508075689,-0.3,0.9));
#17320=CARTESIAN_POINT('',(7.18660254037844,-0.3,0.9));
#17321=CARTESIAN_POINT('',(8.97320508075689,-0.3,0.6));
#17322=CARTESIAN_POINT('',(8.97320508075689,-0.3,0.9));
#17323=CARTESIAN_POINT('',(8.62679491924311,-0.3,0.6));
#17324=CARTESIAN_POINT('Origin',(9.14641016151377,0.,0.9));
#17325=CARTESIAN_POINT('',(8.67810889132456,-0.811121593216771,0.9));
#17326=CARTESIAN_POINT('',(8.97320508075689,-0.3,0.6));
#17327=CARTESIAN_POINT('Origin',(8.8,5.55111512312578E-17,0.6));
#17328=CARTESIAN_POINT('',(8.63,-2.0818995585505E-17,0.6));
#17329=CARTESIAN_POINT('Origin',(8.8,0.,0.6));
#17330=CARTESIAN_POINT('Origin',(2.17320508075689,0.3,0.9));
#17331=CARTESIAN_POINT('',(2.17320508075689,0.3,0.9));
#17332=CARTESIAN_POINT('',(2.34641016151378,0.,0.9));
#17333=CARTESIAN_POINT('',(2.64150635094611,-0.511121593216773,0.9));
#17334=CARTESIAN_POINT('',(2.17320508075689,0.3,0.6));
#17335=CARTESIAN_POINT('',(2.17320508075689,0.3,0.9));
#17336=CARTESIAN_POINT('',(2.34641016151378,0.,0.6));
#17337=CARTESIAN_POINT('',(2.34641016151378,0.,0.6));
#17338=CARTESIAN_POINT('',(2.34641016151378,0.,0.9));
#17339=CARTESIAN_POINT('Origin',(1.82679491924311,0.3,0.9));
#17340=CARTESIAN_POINT('',(1.82679491924311,0.3,0.9));
#17341=CARTESIAN_POINT('',(3.61339745962156,0.3,0.9));
#17342=CARTESIAN_POINT('',(1.82679491924311,0.3,0.6));
#17343=CARTESIAN_POINT('',(1.82679491924311,0.3,0.9));
#17344=CARTESIAN_POINT('',(2.17320508075689,0.3,0.6));
#17345=CARTESIAN_POINT('Origin',(1.65358983848622,5.55111512312578E-17,
0.9));
#17346=CARTESIAN_POINT('',(1.65358983848622,4.24230095489963E-17,0.9));
#17347=CARTESIAN_POINT('',(2.12189110867545,0.811121593216773,0.9));
#17348=CARTESIAN_POINT('',(1.65358983848622,5.55111512312578E-17,0.6));
#17349=CARTESIAN_POINT('',(1.65358983848622,4.24230095489963E-17,0.9));
#17350=CARTESIAN_POINT('',(1.82679491924311,0.3,0.6));
#17351=CARTESIAN_POINT('Origin',(1.82679491924311,-0.3,0.9));
#17352=CARTESIAN_POINT('',(1.82679491924311,-0.3,0.9));
#17353=CARTESIAN_POINT('',(2.20849364905389,-0.961121593216772,0.9));
#17354=CARTESIAN_POINT('',(1.82679491924311,-0.3,0.6));
#17355=CARTESIAN_POINT('',(1.82679491924311,-0.3,0.9));
#17356=CARTESIAN_POINT('',(1.65358983848622,4.24230095489963E-17,0.6));
#17357=CARTESIAN_POINT('Origin',(2.17320508075689,-0.3,0.9));
#17358=CARTESIAN_POINT('',(2.17320508075689,-0.3,0.9));
#17359=CARTESIAN_POINT('',(3.78660254037844,-0.3,0.9));
#17360=CARTESIAN_POINT('',(2.17320508075689,-0.3,0.6));
#17361=CARTESIAN_POINT('',(2.17320508075689,-0.3,0.9));
#17362=CARTESIAN_POINT('',(1.82679491924311,-0.3,0.6));
#17363=CARTESIAN_POINT('Origin',(2.34641016151378,0.,0.9));
#17364=CARTESIAN_POINT('',(2.72810889132455,0.661121593216773,0.9));
#17365=CARTESIAN_POINT('',(2.17320508075689,-0.3,0.6));
#17366=CARTESIAN_POINT('Origin',(2.,5.55111512312578E-17,0.6));
#17367=CARTESIAN_POINT('',(1.83,-2.0818995585505E-17,0.6));
#17368=CARTESIAN_POINT('Origin',(2.,0.,0.6));
#17369=CARTESIAN_POINT('Origin',(8.1,-1.,0.8));
#17370=CARTESIAN_POINT('',(7.95,-1.,0.9));
#17371=CARTESIAN_POINT('Origin',(8.1,-1.,0.9));
#17372=CARTESIAN_POINT('',(7.95,-1.,0.8));
#17373=CARTESIAN_POINT('Origin',(2.7,-1.,0.8));
#17374=CARTESIAN_POINT('',(2.55,-1.,0.9));
#17375=CARTESIAN_POINT('Origin',(2.7,-1.,0.9));
#17376=CARTESIAN_POINT('',(2.55,-1.,0.7));
#17377=CARTESIAN_POINT('',(2.55,-1.,0.8));
#17378=CARTESIAN_POINT('Origin',(2.7,-1.,0.7));
#17379=CARTESIAN_POINT('Origin',(2.7,1.,0.8));
#17380=CARTESIAN_POINT('',(2.55,1.,0.9));
#17381=CARTESIAN_POINT('Origin',(2.7,1.,0.9));
#17382=CARTESIAN_POINT('',(2.55,1.,0.7));
#17383=CARTESIAN_POINT('',(2.55,1.,0.8));
#17384=CARTESIAN_POINT('Origin',(2.7,1.,0.7));
#17385=CARTESIAN_POINT('Origin',(8.1,1.,0.8));
#17386=CARTESIAN_POINT('',(7.95,1.,0.9));
#17387=CARTESIAN_POINT('Origin',(8.1,1.,0.9));
#17388=CARTESIAN_POINT('',(7.95,1.,0.8));
#17389=CARTESIAN_POINT('Origin',(2.,0.,0.45));
#17390=CARTESIAN_POINT('',(1.83,-2.0818995585505E-17,0.32));
#17391=CARTESIAN_POINT('',(1.83,2.0818995585505E-17,0.45));
#17392=CARTESIAN_POINT('Origin',(2.,0.,0.32));
#17393=CARTESIAN_POINT('Origin',(8.8,0.,0.45));
#17394=CARTESIAN_POINT('',(8.63,-2.0818995585505E-17,0.32));
#17395=CARTESIAN_POINT('',(8.63,2.0818995585505E-17,0.45));
#17396=CARTESIAN_POINT('Origin',(8.8,0.,0.32));
#17397=CARTESIAN_POINT('Origin',(10.,-0.62,0.32));
#17398=CARTESIAN_POINT('',(0.200274469199584,-0.62,0.));
#17399=CARTESIAN_POINT('',(0.217044958570157,-0.62,0.32));
#17400=CARTESIAN_POINT('',(0.221783445591644,-0.62,0.410415718550007));
#17401=CARTESIAN_POINT('',(0.,-0.62,0.));
#17402=CARTESIAN_POINT('',(7.7,-0.62,0.));
#17403=CARTESIAN_POINT('',(0.0167704893705732,-0.62,0.32));
#17404=CARTESIAN_POINT('',(0.0220575386407278,-0.62,0.420882909798596));
#17405=CARTESIAN_POINT('',(-0.1,-0.62,0.32));
#17406=CARTESIAN_POINT('Origin',(10.,-0.62,0.32));
#17407=CARTESIAN_POINT('',(0.9,-0.62,0.32));
#17408=CARTESIAN_POINT('',(0.9,-0.62,0.));
#17409=CARTESIAN_POINT('',(0.9,-0.62,0.16));
#17410=CARTESIAN_POINT('',(1.1,-0.62,0.32));
#17411=CARTESIAN_POINT('',(-0.1,-0.62,0.32));
#17412=CARTESIAN_POINT('',(1.1,-0.62,0.));
#17413=CARTESIAN_POINT('',(1.1,-0.62,0.16));
#17414=CARTESIAN_POINT('',(7.7,-0.62,0.));
#17415=CARTESIAN_POINT('Origin',(10.,-0.62,0.32));
#17416=CARTESIAN_POINT('',(3.5,-0.62,0.32));
#17417=CARTESIAN_POINT('',(3.5,-0.62,0.));
#17418=CARTESIAN_POINT('',(3.5,-0.62,0.16));
#17419=CARTESIAN_POINT('',(3.7,-0.62,0.32));
#17420=CARTESIAN_POINT('',(-0.1,-0.62,0.32));
#17421=CARTESIAN_POINT('',(3.7,-0.62,0.));
#17422=CARTESIAN_POINT('',(3.7,-0.62,0.16));
#17423=CARTESIAN_POINT('',(7.7,-0.62,0.));
#17424=CARTESIAN_POINT('Origin',(10.,-0.62,0.32));
#17425=CARTESIAN_POINT('',(7.1,-0.62,0.32));
#17426=CARTESIAN_POINT('',(7.1,-0.62,0.));
#17427=CARTESIAN_POINT('',(7.1,-0.62,0.16));
#17428=CARTESIAN_POINT('',(7.3,-0.62,0.32));
#17429=CARTESIAN_POINT('',(-0.1,-0.62,0.32));
#17430=CARTESIAN_POINT('',(7.3,-0.62,0.));
#17431=CARTESIAN_POINT('',(7.3,-0.62,0.16));
#17432=CARTESIAN_POINT('',(7.7,-0.62,0.));
#17433=CARTESIAN_POINT('Origin',(-0.0999999999999996,0.62,0.32));
#17434=CARTESIAN_POINT('',(0.217044958570158,0.62,0.32));
#17435=CARTESIAN_POINT('',(0.200274469199584,0.62,0.));
#17436=CARTESIAN_POINT('',(0.207951231396534,0.62,0.146481348799182));
#17437=CARTESIAN_POINT('',(0.0167704893705736,0.62,0.32));
#17438=CARTESIAN_POINT('',(10.,0.62,0.32));
#17439=CARTESIAN_POINT('',(0.,0.62,0.));
#17440=CARTESIAN_POINT('',(0.00822532444561912,0.62,0.156948540047771));
#17441=CARTESIAN_POINT('',(2.65,0.62,0.));
#17442=CARTESIAN_POINT('Origin',(-0.0999999999999996,0.62,0.32));
#17443=CARTESIAN_POINT('',(0.9,0.62,0.));
#17444=CARTESIAN_POINT('',(0.9,0.62,0.32));
#17445=CARTESIAN_POINT('',(0.9,0.62,0.16));
#17446=CARTESIAN_POINT('',(1.1,0.62,0.));
#17447=CARTESIAN_POINT('',(2.65,0.62,0.));
#17448=CARTESIAN_POINT('',(1.1,0.62,0.32));
#17449=CARTESIAN_POINT('',(1.1,0.62,0.16));
#17450=CARTESIAN_POINT('',(10.,0.62,0.32));
#17451=CARTESIAN_POINT('Origin',(-0.0999999999999996,0.62,0.32));
#17452=CARTESIAN_POINT('',(3.5,0.62,0.));
#17453=CARTESIAN_POINT('',(3.5,0.62,0.32));
#17454=CARTESIAN_POINT('',(3.5,0.62,0.16));
#17455=CARTESIAN_POINT('',(3.7,0.62,0.));
#17456=CARTESIAN_POINT('',(2.65,0.62,0.));
#17457=CARTESIAN_POINT('',(3.7,0.62,0.32));
#17458=CARTESIAN_POINT('',(3.7,0.62,0.16));
#17459=CARTESIAN_POINT('',(10.,0.62,0.32));
#17460=CARTESIAN_POINT('Origin',(4.95,0.,0.32));
#17461=CARTESIAN_POINT('',(1.6,-4.89858719658941E-17,0.32));
#17462=CARTESIAN_POINT('Origin',(2.,0.,0.32));
#17463=CARTESIAN_POINT('Origin',(4.95,0.,0.32));
#17464=CARTESIAN_POINT('',(8.4,-4.89858719658942E-17,0.32));
#17465=CARTESIAN_POINT('Origin',(8.8,0.,0.32));
#17466=CARTESIAN_POINT('Origin',(4.95,0.,0.32));
#17467=CARTESIAN_POINT('',(0.217044958570157,-0.7,0.32));
#17468=CARTESIAN_POINT('',(0.0167704893705731,-0.7,0.32));
#17469=CARTESIAN_POINT('Origin',(4.95,0.,0.32));
#17470=CARTESIAN_POINT('',(0.9,0.671641708581009,0.32));
#17471=CARTESIAN_POINT('',(1.1,-0.671641708581009,0.32));
#17472=CARTESIAN_POINT('Origin',(4.95,0.,0.32));
#17473=CARTESIAN_POINT('',(3.5,0.723888888888889,0.32));
#17474=CARTESIAN_POINT('',(3.7,-0.723888888888889,0.32));
#17475=CARTESIAN_POINT('Origin',(4.95,0.,0.32));
#17476=CARTESIAN_POINT('',(7.1,0.62,0.32));
#17477=CARTESIAN_POINT('',(7.1,0.712777777777778,0.32));
#17478=CARTESIAN_POINT('',(7.3,0.62,0.32));
#17479=CARTESIAN_POINT('',(10.,0.62,0.32));
#17480=CARTESIAN_POINT('',(7.3,-0.712777777777778,0.32));
#17481=CARTESIAN_POINT('Origin',(-0.0999999999999996,0.62,0.32));
#17482=CARTESIAN_POINT('',(7.1,0.62,0.));
#17483=CARTESIAN_POINT('',(7.1,0.62,0.16));
#17484=CARTESIAN_POINT('',(7.3,0.62,0.));
#17485=CARTESIAN_POINT('',(2.65,0.62,0.));
#17486=CARTESIAN_POINT('',(7.3,0.62,0.16));
#17487=CARTESIAN_POINT('Origin',(10.,1.30754691548544,0.));
#17488=CARTESIAN_POINT('',(10.,1.24211782565704,0.));
#17489=CARTESIAN_POINT('',(10.,-1.24211782565704,0.));
#17490=CARTESIAN_POINT('',(10.,1.30754691548544,0.));
#17491=CARTESIAN_POINT('',(10.,-1.20899340483173,0.605457329065657));
#17492=CARTESIAN_POINT('Ctrl Pts',(10.,-1.20899340483173,0.605457329065657));
#17493=CARTESIAN_POINT('Ctrl Pts',(10.,-1.21451837038612,0.504502771559899));
#17494=CARTESIAN_POINT('Ctrl Pts',(10.,-1.22004249263249,0.403547366186347));
#17495=CARTESIAN_POINT('Ctrl Pts',(10.,-1.23108392958594,0.201728789021226));
#17496=CARTESIAN_POINT('Ctrl Pts',(10.,-1.23660133320922,0.100864020914724));
#17497=CARTESIAN_POINT('Ctrl Pts',(10.,-1.24211782565704,0.));
#17498=CARTESIAN_POINT('Ctrl Pts',(10.,-1.10900986674273,0.7));
#17499=CARTESIAN_POINT('Ctrl Pts',(10.,-1.11692706738765,0.7));
#17500=CARTESIAN_POINT('Ctrl Pts',(9.99999896020971,-1.12478097169818,0.699006158364426));
#17501=CARTESIAN_POINT('Ctrl Pts',(9.99999805494427,-1.13243115645175,0.697118998397561));
#17502=CARTESIAN_POINT('Ctrl Pts',(9.99999754769332,-1.13671781459207,0.696061558623929));
#17503=CARTESIAN_POINT('Ctrl Pts',(9.99999708556116,-1.14094056283945,0.694722610426682));
#17504=CARTESIAN_POINT('Ctrl Pts',(9.99999679002998,-1.14507302265453,0.693112977943955));
#17505=CARTESIAN_POINT('Ctrl Pts',(9.99999625879002,-1.15250143622127,0.690219540062595));
#17506=CARTESIAN_POINT('Ctrl Pts',(9.999996365957,-1.15955821040664,0.686485807665162));
#17507=CARTESIAN_POINT('Ctrl Pts',(9.99999703387985,-1.16609707610076,0.681992895329386));
#17508=CARTESIAN_POINT('Ctrl Pts',(9.99999740034986,-1.16968476316425,0.679527763880215));
#17509=CARTESIAN_POINT('Ctrl Pts',(9.99999792190556,-1.17311627083768,0.676833210412541));
#17510=CARTESIAN_POINT('Ctrl Pts',(9.99999838578331,-1.17636354905877,0.673917165661822));
#17511=CARTESIAN_POINT('Ctrl Pts',(9.99999884023993,-1.17954487655573,0.671060344436104));
#17512=CARTESIAN_POINT('Ctrl Pts',(9.99999924462882,-1.18253006594632,0.668008218820746));
#17513=CARTESIAN_POINT('Ctrl Pts',(9.99999924442301,-1.185296421281,0.664772262763763));
#17514=CARTESIAN_POINT('Ctrl Pts',(9.99999924404215,-1.19041578560695,0.658783864313737));
#17515=CARTESIAN_POINT('Ctrl Pts',(9.99999800949836,-1.19478865237554,0.652167294255586));
#17516=CARTESIAN_POINT('Ctrl Pts',(9.99999759228052,-1.19835462180986,0.645087621913151));
#17517=CARTESIAN_POINT('Ctrl Pts',(9.99999755030119,-1.19871341999785,0.644375284453517));
#17518=CARTESIAN_POINT('Ctrl Pts',(9.9999975145836,-1.19906401030029,0.643658239626438));
#17519=CARTESIAN_POINT('Ctrl Pts',(9.99999748581823,-1.19940630408966,0.642936645100882));
#17520=CARTESIAN_POINT('Ctrl Pts',(9.99999720003888,-1.20280693749908,0.635767720253638));
#17521=CARTESIAN_POINT('Ctrl Pts',(9.9999978299417,-1.20535324884233,0.628234501710241));
#17522=CARTESIAN_POINT('Ctrl Pts',(9.99999874867777,-1.20699142055415,0.62050509267719));
#17523=CARTESIAN_POINT('Ctrl Pts',(9.99999933690345,-1.20804026874419,0.615556297251186));
#17524=CARTESIAN_POINT('Ctrl Pts',(9.99999999916487,-1.20871598809812,0.61052641213707));
#17525=CARTESIAN_POINT('Ctrl Pts',(9.99999999968202,-1.20899340489109,0.605457329065633));
#17526=CARTESIAN_POINT('Ctrl Pts',(10.,1.24211782565704,0.));
#17527=CARTESIAN_POINT('Ctrl Pts',(10.,1.23660053043673,0.100878698875723));
#17528=CARTESIAN_POINT('Ctrl Pts',(10.,1.23108232376984,0.201758145268796));
#17529=CARTESIAN_POINT('Ctrl Pts',(10.,1.22004088630648,0.403576722396156));
#17530=CARTESIAN_POINT('Ctrl Pts',(10.,1.2145175671044,0.504517449470448));
#17531=CARTESIAN_POINT('Ctrl Pts',(10.,1.20899340483173,0.605457329065657));
#17532=CARTESIAN_POINT('Origin',(7.3,-1.42555555555556,0.));
#17533=CARTESIAN_POINT('',(7.3,1.35236351479115,0.));
#17534=CARTESIAN_POINT('',(7.3,-1.42555555555556,0.));
#17535=CARTESIAN_POINT('Ctrl Pts',(7.29999999953133,1.3203161347307,0.605285370449834));
#17536=CARTESIAN_POINT('Ctrl Pts',(7.29999999953133,1.32565322760551,0.504490726585133));
#17537=CARTESIAN_POINT('Ctrl Pts',(7.3,1.33099015509697,0.403695123734478));
#17538=CARTESIAN_POINT('Ctrl Pts',(7.3,1.34167258064689,0.201933969199042));
#17539=CARTESIAN_POINT('Ctrl Pts',(7.3,1.34701817868136,0.100966514951419));
#17540=CARTESIAN_POINT('Ctrl Pts',(7.3,1.35236351479115,0.));
#17541=CARTESIAN_POINT('',(7.29999999953133,-1.3203161347307,0.605285370449834));
#17542=CARTESIAN_POINT('Ctrl Pts',(7.3,-1.32031613470337,0.605285370449877));
#17543=CARTESIAN_POINT('Ctrl Pts',(7.3,-1.31989712778929,0.61319860217968));
#17544=CARTESIAN_POINT('Ctrl Pts',(7.29999916171872,-1.31851071739963,0.621020829077898));
#17545=CARTESIAN_POINT('Ctrl Pts',(7.29999878808195,-1.31624092632926,0.628591660945423));
#17546=CARTESIAN_POINT('Ctrl Pts',(7.29999857947278,-1.31497365483497,0.632818613610392));
#17547=CARTESIAN_POINT('Ctrl Pts',(7.29999848639856,-1.31343001415,0.636967235874856));
#17548=CARTESIAN_POINT('Ctrl Pts',(7.29999853830689,-1.31161789606625,0.641007613679984));
#17549=CARTESIAN_POINT('Ctrl Pts',(7.29999863125487,-1.30837308502546,0.648242386418365));
#17550=CARTESIAN_POINT('Ctrl Pts',(7.29999925734287,-1.30430566789097,0.655052076019481));
#17551=CARTESIAN_POINT('Ctrl Pts',(7.29999949821933,-1.29947941328181,0.661273460789274));
#17552=CARTESIAN_POINT('Ctrl Pts',(7.29999954322,-1.29857776968225,0.662435743389828));
#17553=CARTESIAN_POINT('Ctrl Pts',(7.29999957102613,-1.29764951297213,0.663577423078133));
#17554=CARTESIAN_POINT('Ctrl Pts',(7.2999995707084,-1.29669488998092,0.664697318929248));
#17555=CARTESIAN_POINT('Ctrl Pts',(7.29999957007561,-1.29479368240016,0.666927680549918));
#17556=CARTESIAN_POINT('Ctrl Pts',(7.29999945886743,-1.29278792931167,0.669071688571899));
#17557=CARTESIAN_POINT('Ctrl Pts',(7.29999930790078,-1.2906849717248,0.671125563583336));
#17558=CARTESIAN_POINT('Ctrl Pts',(7.29999889984047,-1.28500071247856,0.676677153447665));
#17559=CARTESIAN_POINT('Ctrl Pts',(7.29999826931494,-1.27867319504519,0.681510485910933));
#17560=CARTESIAN_POINT('Ctrl Pts',(7.29999806345125,-1.27186607945067,0.685571085769401));
#17561=CARTESIAN_POINT('Ctrl Pts',(7.29999793266427,-1.26754145993833,0.688150820039508));
#17562=CARTESIAN_POINT('Ctrl Pts',(7.29999794545359,-1.26302231037287,0.690417984675215));
#17563=CARTESIAN_POINT('Ctrl Pts',(7.29999810371711,-1.25834494218995,0.69234933099425));
#17564=CARTESIAN_POINT('Ctrl Pts',(7.29999835129001,-1.25102809722258,0.695370551698293));
#17565=CARTESIAN_POINT('Ctrl Pts',(7.29999895574222,-1.24340909242398,0.6975375590939));
#17566=CARTESIAN_POINT('Ctrl Pts',(7.29999944081525,-1.2356348173965,0.698780605629559));
#17567=CARTESIAN_POINT('Ctrl Pts',(7.29999975409932,-1.23061380764338,0.699583426311495));
#17568=CARTESIAN_POINT('Ctrl Pts',(7.30000000047446,-1.22552743956586,0.699999999832051));
#17569=CARTESIAN_POINT('Ctrl Pts',(7.29999999989087,-1.22041345054982,0.7));
#17570=CARTESIAN_POINT('',(7.3,-1.35236351479115,0.));
#17571=CARTESIAN_POINT('Ctrl Pts',(7.3,-1.35236351479115,0.));
#17572=CARTESIAN_POINT('Ctrl Pts',(7.3,-1.34701814920095,0.100967071798286));
#17573=CARTESIAN_POINT('Ctrl Pts',(7.3,-1.34167252169398,0.201935082699409));
#17574=CARTESIAN_POINT('Ctrl Pts',(7.3,-1.33099009614589,0.403696237111114));
#17575=CARTESIAN_POINT('Ctrl Pts',(7.29999999953133,-1.32565319812959,0.504491283257837));
#17576=CARTESIAN_POINT('Ctrl Pts',(7.29999999953133,-1.3203161347307,0.605285370449834));
#17577=CARTESIAN_POINT('',(7.3,-1.42555555555556,0.));
#17578=CARTESIAN_POINT('Origin',(3.7,-1.44777777777778,0.));
#17579=CARTESIAN_POINT('',(3.7,1.37924639543935,0.));
#17580=CARTESIAN_POINT('',(3.7,-1.44777777777778,0.));
#17581=CARTESIAN_POINT('',(3.7,1.34735368793805,0.605261457205193));
#17582=CARTESIAN_POINT('Ctrl Pts',(3.7,1.34735368793805,0.605261457205193));
#17583=CARTESIAN_POINT('Ctrl Pts',(3.7,1.35266395147774,0.504488703431434));
#17584=CARTESIAN_POINT('Ctrl Pts',(3.7,1.35797406404029,0.40371594170176));
#17585=CARTESIAN_POINT('Ctrl Pts',(3.7,1.36860496587027,0.201962122597264));
#17586=CARTESIAN_POINT('Ctrl Pts',(3.7,1.37392575452088,0.100981065191366));
#17587=CARTESIAN_POINT('Ctrl Pts',(3.7,1.37924639543935,0.));
#17588=CARTESIAN_POINT('',(3.7,1.24747724070879,0.7));
#17589=CARTESIAN_POINT('Ctrl Pts',(3.7,1.24747724070879,0.7));
#17590=CARTESIAN_POINT('Ctrl Pts',(3.7,1.25538532734776,0.7));
#17591=CARTESIAN_POINT('Ctrl Pts',(3.70000034866643,1.26322972530331,0.699006048248363));
#17592=CARTESIAN_POINT('Ctrl Pts',(3.70000065268588,1.27087026624727,0.697119044026295));
#17593=CARTESIAN_POINT('Ctrl Pts',(3.7000008238479,1.27517186762995,0.696056666371322));
#17594=CARTESIAN_POINT('Ctrl Pts',(3.70000097972585,1.27940891103121,0.694710185093394));
#17595=CARTESIAN_POINT('Ctrl Pts',(3.70000107833511,1.28355469746902,0.693090631030141));
#17596=CARTESIAN_POINT('Ctrl Pts',(3.70000125487464,1.29097687270382,0.690191153635441));
#17597=CARTESIAN_POINT('Ctrl Pts',(3.7000012145424,1.29802606517866,0.686451118058958));
#17598=CARTESIAN_POINT('Ctrl Pts',(3.70000098691147,1.3045562506385,0.681952404110064));
#17599=CARTESIAN_POINT('Ctrl Pts',(3.70000086156653,1.30815209635338,0.679475187900035));
#17600=CARTESIAN_POINT('Ctrl Pts',(3.70000068390876,1.31159030769532,0.676767042898431));
#17601=CARTESIAN_POINT('Ctrl Pts',(3.70000052608992,1.31484259178137,0.673836088143417));
#17602=CARTESIAN_POINT('Ctrl Pts',(3.70000037216713,1.31801458722906,0.670977489418868));
#17603=CARTESIAN_POINT('Ctrl Pts',(3.70000023558528,1.32099045552882,0.667924239810466));
#17604=CARTESIAN_POINT('Ctrl Pts',(3.70000023595245,1.32374763345498,0.664687876924229));
#17605=CARTESIAN_POINT('Ctrl Pts',(3.70000023663259,1.32885491153898,0.658692977181302));
#17606=CARTESIAN_POINT('Ctrl Pts',(3.70000065621025,1.33321474659758,0.652071180203097));
#17607=CARTESIAN_POINT('Ctrl Pts',(3.70000080093706,1.33676785491319,0.644988218508662));
#17608=CARTESIAN_POINT('Ctrl Pts',(3.70000081573428,1.33713113341147,0.644264039153811));
#17609=CARTESIAN_POINT('Ctrl Pts',(3.70000082835625,1.33748593861467,0.643535019157411));
#17610=CARTESIAN_POINT('Ctrl Pts',(3.70000083855542,1.33783217873901,0.642801324492746));
#17611=CARTESIAN_POINT('Ctrl Pts',(3.70000093832019,1.34121897990539,0.63562457699476));
#17612=CARTESIAN_POINT('Ctrl Pts',(3.70000072997693,1.34375116782692,0.628085030530103));
#17613=CARTESIAN_POINT('Ctrl Pts',(3.70000042189378,1.34537558692779,0.6203512574804));
#17614=CARTESIAN_POINT('Ctrl Pts',(3.70000022417294,1.3464181026242,0.615387895628485));
#17615=CARTESIAN_POINT('Ctrl Pts',(3.70000000036652,1.34708586836718,0.6103438638189));
#17616=CARTESIAN_POINT('Ctrl Pts',(3.69999999992214,1.34735368792773,0.6052614572053));
#17617=CARTESIAN_POINT('',(3.7,-1.24747724070944,0.7));
#17618=CARTESIAN_POINT('',(3.7,-0.723888888888889,0.7));
#17619=CARTESIAN_POINT('',(3.7,-1.34735368793805,0.605261457205193));
#17620=CARTESIAN_POINT('Ctrl Pts',(3.69999999992215,-1.34735368792773,0.6052614572053));
#17621=CARTESIAN_POINT('Ctrl Pts',(3.70000000061408,-1.34693666923469,0.613175212866596));
#17622=CARTESIAN_POINT('Ctrl Pts',(3.70000049671034,-1.34555248374866,0.620998392122869));
#17623=CARTESIAN_POINT('Ctrl Pts',(3.70000071566022,-1.34328499565267,0.628570462735333));
#17624=CARTESIAN_POINT('Ctrl Pts',(3.70000083807517,-1.34201724238155,0.632804009674372));
#17625=CARTESIAN_POINT('Ctrl Pts',(3.7000008913247,-1.34047237297042,0.63695909738719));
#17626=CARTESIAN_POINT('Ctrl Pts',(3.70000085837557,-1.33865827982058,0.641005656934072));
#17627=CARTESIAN_POINT('Ctrl Pts',(3.7000007994669,-1.33541492172585,0.648240369034365));
#17628=CARTESIAN_POINT('Ctrl Pts',(3.70000042420685,-1.33134915897915,0.655050234746405));
#17629=CARTESIAN_POINT('Ctrl Pts',(3.70000027984635,-1.32652447879733,0.661271863919233));
#17630=CARTESIAN_POINT('Ctrl Pts',(3.70000025294096,-1.32562527203035,0.662431429080655));
#17631=CARTESIAN_POINT('Ctrl Pts',(3.7000002362737,-1.32469957579387,0.663570491348455));
#17632=CARTESIAN_POINT('Ctrl Pts',(3.70000023630138,-1.32374763346102,0.664687876924223));
#17633=CARTESIAN_POINT('Ctrl Pts',(3.70000023635686,-1.32184039796576,0.666926581264246));
#17634=CARTESIAN_POINT('Ctrl Pts',(3.70000030283857,-1.31982784222224,0.669078323867587));
#17635=CARTESIAN_POINT('Ctrl Pts',(3.70000039320883,-1.31771738411303,0.671139279696989));
#17636=CARTESIAN_POINT('Ctrl Pts',(3.70000063660146,-1.3120333248939,0.676690015307994));
#17637=CARTESIAN_POINT('Ctrl Pts',(3.7000010126336,-1.30570602994251,0.681522474044465));
#17638=CARTESIAN_POINT('Ctrl Pts',(3.70000113724274,-1.29889910811053,0.685582059356066));
#17639=CARTESIAN_POINT('Ctrl Pts',(3.70000121634872,-1.29457784995583,0.688159217808216));
#17640=CARTESIAN_POINT('Ctrl Pts',(3.70000121058612,-1.2900623422215,0.690424215862126));
#17641=CARTESIAN_POINT('Ctrl Pts',(3.70000111831253,-1.28538881676413,0.692353818784707));
#17642=CARTESIAN_POINT('Ctrl Pts',(3.70000097388434,-1.27807373536961,0.695374066040565));
#17643=CARTESIAN_POINT('Ctrl Pts',(3.70000061691996,-1.27045659963863,0.697540160564298));
#17644=CARTESIAN_POINT('Ctrl Pts',(3.7000003304055,-1.26268427129293,0.698782316368755));
#17645=CARTESIAN_POINT('Ctrl Pts',(3.70000014548661,-1.25766794365683,0.699584014420239));
#17646=CARTESIAN_POINT('Ctrl Pts',(3.7,-1.25258637988459,0.7));
#17647=CARTESIAN_POINT('Ctrl Pts',(3.7,-1.24747724070879,0.7));
#17648=CARTESIAN_POINT('',(3.7,-1.37924639543935,0.));
#17649=CARTESIAN_POINT('Ctrl Pts',(3.7,-1.37924639543935,0.));
#17650=CARTESIAN_POINT('Ctrl Pts',(3.7,-1.37392574223662,0.100981298335747));
#17651=CARTESIAN_POINT('Ctrl Pts',(3.7,-1.36860494130098,0.201962588887634));
#17652=CARTESIAN_POINT('Ctrl Pts',(3.7,-1.35797403946962,0.403716407992068));
#17653=CARTESIAN_POINT('Ctrl Pts',(3.7,-1.3526639391921,0.504488936575732));
#17654=CARTESIAN_POINT('Ctrl Pts',(3.7,-1.34735368793805,0.605261457205193));
#17655=CARTESIAN_POINT('',(3.7,-1.44777777777778,0.));
#17656=CARTESIAN_POINT('Origin',(1.1,-1.34328341716202,0.));
#17657=CARTESIAN_POINT('',(1.1,1.27885335043294,0.));
#17658=CARTESIAN_POINT('',(1.1,-1.34328341716202,0.));
#17659=CARTESIAN_POINT('Ctrl Pts',(1.1,1.24553911298206,0.605485603995113));
#17660=CARTESIAN_POINT('Ctrl Pts',(1.1,1.25109559382646,0.504544105903265));
#17661=CARTESIAN_POINT('Ctrl Pts',(1.1,1.25665083308595,0.403601248768354));
#17662=CARTESIAN_POINT('Ctrl Pts',(1.1,1.26775551906787,0.201773573764085));
#17663=CARTESIAN_POINT('Ctrl Pts',(1.1,1.2733051088238,0.100886182270816));
#17664=CARTESIAN_POINT('Ctrl Pts',(1.1,1.27885335043294,0.));
#17665=CARTESIAN_POINT('',(1.1,-1.14549341399195,0.7));
#17666=CARTESIAN_POINT('',(1.1,-0.671641708581009,0.7));
#17667=CARTESIAN_POINT('',(1.1,-1.24553911298206,0.605485603995113));
#17668=CARTESIAN_POINT('Ctrl Pts',(1.09999999916631,-1.24553911263843,0.605485603997431));
#17669=CARTESIAN_POINT('Ctrl Pts',(1.10000000220634,-1.24510362317222,0.61339691285734));
#17670=CARTESIAN_POINT('Ctrl Pts',(1.10000177015643,-1.24370036622144,0.621215229994996));
#17671=CARTESIAN_POINT('Ctrl Pts',(1.10000252895322,-1.24141353486351,0.628780213666851));
#17672=CARTESIAN_POINT('Ctrl Pts',(1.10000294802756,-1.24015054543059,0.632958263090869));
#17673=CARTESIAN_POINT('Ctrl Pts',(1.10000312162076,-1.23861706177488,0.637059070655947));
#17674=CARTESIAN_POINT('Ctrl Pts',(1.10000299297862,-1.23682078380192,0.641053713130525));
#17675=CARTESIAN_POINT('Ctrl Pts',(1.10000275999609,-1.23356756237267,0.64828837095969));
#17676=CARTESIAN_POINT('Ctrl Pts',(1.10000138715103,-1.22949085733774,0.655096441442141));
#17677=CARTESIAN_POINT('Ctrl Pts',(1.10000084482056,-1.2246552743941,0.661315040399663));
#17678=CARTESIAN_POINT('Ctrl Pts',(1.10000074196669,-1.22373819809959,0.662494407966206));
#17679=CARTESIAN_POINT('Ctrl Pts',(1.1000006773267,-1.22279369438101,0.663652502541609));
#17680=CARTESIAN_POINT('Ctrl Pts',(1.10000067553493,-1.22182202641035,0.66478809188211));
#17681=CARTESIAN_POINT('Ctrl Pts',(1.10000067210542,-1.219962222636,0.666961646435043));
#17682=CARTESIAN_POINT('Ctrl Pts',(1.10000089707048,-1.21800293160495,0.669052796220007));
#17683=CARTESIAN_POINT('Ctrl Pts',(1.10000120920309,-1.21595100691259,0.671058078730413));
#17684=CARTESIAN_POINT('Ctrl Pts',(1.10000207391986,-1.21026645613745,0.676613414309409));
#17685=CARTESIAN_POINT('Ctrl Pts',(1.1000034579227,-1.20393786500476,0.681450029097565));
#17686=CARTESIAN_POINT('Ctrl Pts',(1.10000394126019,-1.19712964857754,0.685514663758263));
#17687=CARTESIAN_POINT('Ctrl Pts',(1.10000424974863,-1.19278432848208,0.688108902478585));
#17688=CARTESIAN_POINT('Ctrl Pts',(1.10000425197701,-1.18824265871575,0.690387991283085));
#17689=CARTESIAN_POINT('Ctrl Pts',(1.10000394032285,-1.18354156621637,0.692328715646671));
#17690=CARTESIAN_POINT('Ctrl Pts',(1.10000345443802,-1.17621232165581,0.695354404566264));
#17691=CARTESIAN_POINT('Ctrl Pts',(1.10000219938511,-1.16858027633095,0.697525330589554));
#17692=CARTESIAN_POINT('Ctrl Pts',(1.10000118192936,-1.16079305972554,0.698772417158578));
#17693=CARTESIAN_POINT('Ctrl Pts',(1.10000052251962,-1.15574619011492,0.699580649884844));
#17694=CARTESIAN_POINT('Ctrl Pts',(1.1,-1.15063354328712,0.7));
#17695=CARTESIAN_POINT('Ctrl Pts',(1.1,-1.14549341399196,0.7));
#17696=CARTESIAN_POINT('',(1.1,-1.27885335043294,0.));
#17697=CARTESIAN_POINT('Ctrl Pts',(1.1,-1.27885335043294,0.));
#17698=CARTESIAN_POINT('Ctrl Pts',(1.1,-1.27330503870861,0.100887457206881));
#17699=CARTESIAN_POINT('Ctrl Pts',(1.1,-1.26775537880223,0.201776123688554));
#17700=CARTESIAN_POINT('Ctrl Pts',(1.1,-1.25665069275548,0.403603798678134));
#17701=CARTESIAN_POINT('Ctrl Pts',(1.1,-1.25109552364596,0.504545380833391));
#17702=CARTESIAN_POINT('Ctrl Pts',(1.1,-1.24553911298206,0.605485603995113));
#17703=CARTESIAN_POINT('',(1.1,-1.34328341716202,0.));
#17704=CARTESIAN_POINT('Origin',(0.199725906950915,-1.4,-0.0104671912485888));
#17705=CARTESIAN_POINT('',(0.200274469199584,1.12301388185427,1.38777878078145E-17));
#17706=CARTESIAN_POINT('',(0.200274469199585,-0.7,0.));
#17707=CARTESIAN_POINT('',(0.231993417893744,1.09142177001972,0.605233595624295));
#17708=CARTESIAN_POINT('Ctrl Pts',(0.200274469199584,1.12301388185427,-2.97071395261028E-17));
#17709=CARTESIAN_POINT('Ctrl Pts',(0.210847451470635,1.11248294808,0.201744519910852));
#17710=CARTESIAN_POINT('Ctrl Pts',(0.22142043436526,1.101952242875,0.403489051720196));
#17711=CARTESIAN_POINT('Ctrl Pts',(0.231993417893744,1.09142177001972,0.605233595624295));
#17712=CARTESIAN_POINT('',(0.231993417893744,-1.09142177001972,0.605233595624295));
#17713=CARTESIAN_POINT('',(0.231993417893744,-0.7,0.605233595624295));
#17714=CARTESIAN_POINT('',(0.200274469199584,-1.12301388185427,-1.38777878078145E-17));
#17715=CARTESIAN_POINT('Ctrl Pts',(0.231993417893744,-1.09142177001972,
0.605233595624295));
#17716=CARTESIAN_POINT('Ctrl Pts',(0.22142043436526,-1.101952242875,0.403489051720196));
#17717=CARTESIAN_POINT('Ctrl Pts',(0.210847451470635,-1.11248294808,0.201744519910852));
#17718=CARTESIAN_POINT('Ctrl Pts',(0.200274469199584,-1.12301388185427,
-4.90059381963448E-17));
#17719=CARTESIAN_POINT('',(0.200274469199585,-0.7,0.));
#17720=CARTESIAN_POINT('Origin',(5.4,-1.11022302462516E-16,0.));
#17721=CARTESIAN_POINT('Ctrl Pts',(7.29999999999999,-1.35236351479115,1.04083408558608E-17));
#17722=CARTESIAN_POINT('Ctrl Pts',(8.20044803681595,-1.32637404707459,3.18306896032855E-8));
#17723=CARTESIAN_POINT('Ctrl Pts',(9.10060048441536,-1.28803709316692,1.03188250195688E-8));
#17724=CARTESIAN_POINT('Ctrl Pts',(10.0000000000405,-1.24211782537639,-8.23328475353175E-12));
#17725=CARTESIAN_POINT('Ctrl Pts',(10.0000000000405,1.24211782537639,-8.23320567538283E-12));
#17726=CARTESIAN_POINT('Ctrl Pts',(9.1006004808701,1.28803709334794,1.03184817085883E-8));
#17727=CARTESIAN_POINT('Ctrl Pts',(8.20044803144508,1.32637404722969,3.18291413954212E-8));
#17728=CARTESIAN_POINT('Ctrl Pts',(7.3,1.35236351479115,4.75121773919879E-17));
#17729=CARTESIAN_POINT('',(7.1,1.35793097395724,0.));
#17730=CARTESIAN_POINT('',(7.1,1.42555555555556,0.));
#17731=CARTESIAN_POINT('Ctrl Pts',(7.1000000000396,1.35793097389613,-4.88924676637329E-12));
#17732=CARTESIAN_POINT('Ctrl Pts',(6.53177385320612,1.37316067096195,3.71763852401782E-9));
#17733=CARTESIAN_POINT('Ctrl Pts',(5.96344379069665,1.38333257666104,-3.82408184804385E-8));
#17734=CARTESIAN_POINT('Ctrl Pts',(5.39512359652123,1.38725406840392,-3.97623797275691E-8));
#17735=CARTESIAN_POINT('Ctrl Pts',(4.82973248928002,1.39115534902226,-4.12760989429076E-8));
#17736=CARTESIAN_POINT('Ctrl Pts',(4.26470859812609,1.38886839226708,1.63957607983357E-8));
#17737=CARTESIAN_POINT('Ctrl Pts',(3.70000000036239,1.37924639538501,-6.25376529969227E-12));
#17738=CARTESIAN_POINT('',(3.5,1.37552980833516,0.));
#17739=CARTESIAN_POINT('',(3.5,1.44777777777778,0.));
#17740=CARTESIAN_POINT('Ctrl Pts',(3.50000000097466,1.37552980835479,1.06251812903579E-15));
#17741=CARTESIAN_POINT('Ctrl Pts',(2.69943075695685,1.35940904975719,2.35366119539541E-7));
#17742=CARTESIAN_POINT('Ctrl Pts',(1.89948254587541,1.32827224396921,2.51300192353997E-7));
#17743=CARTESIAN_POINT('Ctrl Pts',(1.10000000028363,1.27885335028943,-5.13283415455519E-11));
#17744=CARTESIAN_POINT('',(0.9,1.266106713614,0.));
#17745=CARTESIAN_POINT('',(0.9,1.34328341716202,0.));
#17746=CARTESIAN_POINT('',(0.292382661757373,1.22257596919059,0.));
#17747=CARTESIAN_POINT('Ctrl Pts',(0.9,1.266106713614,1.20346441145891E-16));
#17748=CARTESIAN_POINT('Ctrl Pts',(0.697432754539207,1.25280566772398,-2.10387859372414E-8));
#17749=CARTESIAN_POINT('Ctrl Pts',(0.494894520889663,1.23831317328004,3.6654767345328E-12));
#17750=CARTESIAN_POINT('Ctrl Pts',(0.292382661757371,1.22257596919059,2.98331735103528E-16));
#17751=CARTESIAN_POINT('Ctrl Pts',(0.292382661757373,1.22257596919059,2.94902990916057E-17));
#17752=CARTESIAN_POINT('Ctrl Pts',(0.284469747869226,1.22196105627757,-8.65621238729993E-13));
#17753=CARTESIAN_POINT('Ctrl Pts',(0.276673396002317,1.22038240716686,-1.19564355630166E-6));
#17754=CARTESIAN_POINT('Ctrl Pts',(0.269153172408756,1.21792571627104,-1.29137975931779E-6));
#17755=CARTESIAN_POINT('Ctrl Pts',(0.264330998492885,1.21635041859408,-1.35276844214688E-6));
#17756=CARTESIAN_POINT('Ctrl Pts',(0.259622238853914,1.21441292414196,-1.0165784587106E-6));
#17757=CARTESIAN_POINT('Ctrl Pts',(0.255072584042237,1.21212521597766,-4.21167369976509E-7));
#17758=CARTESIAN_POINT('Ctrl Pts',(0.247984787860257,1.20856125126747,5.06409032217246E-7));
#17759=CARTESIAN_POINT('Ctrl Pts',(0.241364979299678,1.20419126978451,2.25366520907849E-6));
#17760=CARTESIAN_POINT('Ctrl Pts',(0.235375785094684,1.19908071490398,1.28723124315333E-6));
#17761=CARTESIAN_POINT('Ctrl Pts',(0.235058634311792,1.19881009144014,1.23605486142058E-6));
#17762=CARTESIAN_POINT('Ctrl Pts',(0.234743258170683,1.19853738091759,1.17639378419006E-6));
#17763=CARTESIAN_POINT('Ctrl Pts',(0.234429683218046,1.19826258967301,1.10742116603597E-6));
#17764=CARTESIAN_POINT('Ctrl Pts',(0.23095881299434,1.19522100506769,3.4398325561458E-7));
#17765=CARTESIAN_POINT('Ctrl Pts',(0.227708211416394,1.19192479473749,-1.52348441667556E-6));
#17766=CARTESIAN_POINT('Ctrl Pts',(0.224692430858345,1.18840300965977,-3.42436181452249E-6));
#17767=CARTESIAN_POINT('Ctrl Pts',(0.219522873151367,1.18236607466387,-6.68278702580898E-6));
#17768=CARTESIAN_POINT('Ctrl Pts',(0.21509942609515,1.17573654654733,-9.78259773483875E-6));
#17769=CARTESIAN_POINT('Ctrl Pts',(0.211478909386775,1.16867548752938,-1.04320859863301E-5));
#17770=CARTESIAN_POINT('Ctrl Pts',(0.20968494559888,1.16517673715679,-1.075390701291E-5));
#17771=CARTESIAN_POINT('Ctrl Pts',(0.208088728862602,1.16157146972622,-1.05358292927083E-5));
#17772=CARTESIAN_POINT('Ctrl Pts',(0.206701335101202,1.15787708229469,-9.83193564179307E-6));
#17773=CARTESIAN_POINT('Ctrl Pts',(0.203919119965097,1.15046852899383,-8.42037994342582E-6));
#17774=CARTESIAN_POINT('Ctrl Pts',(0.202003457218558,1.1427818296106,-4.88542801801716E-6));
#17775=CARTESIAN_POINT('Ctrl Pts',(0.201024541128784,1.13496408391561,-2.30807221316776E-6));
#17776=CARTESIAN_POINT('Ctrl Pts',(0.200529226009753,1.13100843574523,-1.00397341389412E-6));
#17777=CARTESIAN_POINT('Ctrl Pts',(0.200274469344113,1.12701892049093,-1.14168925800036E-11));
#17778=CARTESIAN_POINT('Ctrl Pts',(0.200274469199584,1.12301388185427,-1.43114686768087E-17));
#17779=CARTESIAN_POINT('',(-1.73234772679968E-18,1.12356026268968,4.53319947845445E-20));
#17780=CARTESIAN_POINT('',(0.,-1.4,0.));
#17781=CARTESIAN_POINT('',(0.276326924564679,1.42224670711126,-2.77555756156289E-17));
#17782=CARTESIAN_POINT('Ctrl Pts',(0.276326924564681,1.42224670711126,-1.50920942409982E-16));
#17783=CARTESIAN_POINT('Ctrl Pts',(0.258529852003869,1.4208638358667,-3.32972379743633E-13));
#17784=CARTESIAN_POINT('Ctrl Pts',(0.240927013527826,1.41785398988725,-1.99727536601662E-6));
#17785=CARTESIAN_POINT('Ctrl Pts',(0.223720619657732,1.41333325652174,-2.71091968639774E-6));
#17786=CARTESIAN_POINT('Ctrl Pts',(0.206313289378911,1.40875972999491,-3.432897951005E-6));
#17787=CARTESIAN_POINT('Ctrl Pts',(0.18931019325249,1.40263932318529,-2.78724979559428E-6));
#17788=CARTESIAN_POINT('Ctrl Pts',(0.172932985028856,1.39504220432096,-6.31841720307455E-7));
#17789=CARTESIAN_POINT('Ctrl Pts',(0.170060146426803,1.39370954151055,-2.53746782677961E-7));
#17790=CARTESIAN_POINT('Ctrl Pts',(0.167206630967902,1.39233132643846,1.61597591574489E-7));
#17791=CARTESIAN_POINT('Ctrl Pts',(0.164373729059928,1.39090779908693,6.02790108062464E-7));
#17792=CARTESIAN_POINT('Ctrl Pts',(0.148213121449433,1.38278712717586,3.11962244863226E-6));
#17793=CARTESIAN_POINT('Ctrl Pts',(0.132864864406694,1.37326763401578,6.8005293729143E-6));
#17794=CARTESIAN_POINT('Ctrl Pts',(0.118540368157823,1.36244192017091,7.47011412280372E-6));
#17795=CARTESIAN_POINT('Ctrl Pts',(0.1130124780146,1.35826422653222,7.72851001154276E-6));
#17796=CARTESIAN_POINT('Ctrl Pts',(0.107637267132642,1.35389150739715,7.50091387420595E-6));
#17797=CARTESIAN_POINT('Ctrl Pts',(0.102427993107927,1.34932731552598,6.39696583889361E-6));
#17798=CARTESIAN_POINT('Ctrl Pts',(0.0920147884934566,1.34020361352282,
4.19020214765608E-6));
#17799=CARTESIAN_POINT('Ctrl Pts',(0.082263696775192,1.33031540618347,-1.43705507633734E-6));
#17800=CARTESIAN_POINT('Ctrl Pts',(0.0732179607829324,1.31975004019149,
-7.24116446069057E-6));
#17801=CARTESIAN_POINT('Ctrl Pts',(0.0614369648181435,1.30598990677343,
-1.48003270644599E-5));
#17802=CARTESIAN_POINT('Ctrl Pts',(0.0509520748529884,1.29120077200215,
-2.24515165560165E-5));
#17803=CARTESIAN_POINT('Ctrl Pts',(0.0418305631051555,1.27560026299671,
-2.64881615939377E-5));
#17804=CARTESIAN_POINT('Ctrl Pts',(0.0329966685655992,1.26049166530727,
-3.03975241584371E-5));
#17805=CARTESIAN_POINT('Ctrl Pts',(0.0254411283904758,1.24462062939249,
-3.09701348507133E-5));
#17806=CARTESIAN_POINT('Ctrl Pts',(0.0192647836588538,1.2281607987719,-2.81763116144976E-5));
#17807=CARTESIAN_POINT('Ctrl Pts',(0.0129258683931997,1.2112677210496,-2.53089508159798E-5));
#17808=CARTESIAN_POINT('Ctrl Pts',(0.00809110271874438,1.19389182855556,
-1.89493195503086E-5));
#17809=CARTESIAN_POINT('Ctrl Pts',(0.00484442764459327,1.17622983835018,
-1.25518552566888E-5));
#17810=CARTESIAN_POINT('Ctrl Pts',(0.00165723550742335,1.1588914367474,
-6.27160009448058E-6));
#17811=CARTESIAN_POINT('Ctrl Pts',(1.90718451428807E-9,1.14127598190669,
-1.51296892603399E-10));
#17812=CARTESIAN_POINT('Ctrl Pts',(2.41777084464267E-17,1.12356026268968,
-3.46944695195361E-18));
#17813=CARTESIAN_POINT('',(10.5166159648474,1.4155315881283,0.));
#17814=CARTESIAN_POINT('Ctrl Pts',(0.276326924564679,1.42224670711126,0.));
#17815=CARTESIAN_POINT('Ctrl Pts',(3.68975660465893,1.68747752195839,0.));
#17816=CARTESIAN_POINT('Ctrl Pts',(7.10318628475318,1.599994843061,0.));
#17817=CARTESIAN_POINT('Ctrl Pts',(10.5166159648474,1.4155315881283,0.));
#17818=CARTESIAN_POINT('',(10.8,1.11638029377732,-5.56631991785941E-17));
#17819=CARTESIAN_POINT('Ctrl Pts',(10.8,1.11638029377732,2.32452945780892E-16));
#17820=CARTESIAN_POINT('Ctrl Pts',(10.7999999994302,1.13421844616111,-9.29296349749781E-12));
#17821=CARTESIAN_POINT('Ctrl Pts',(10.7983603663884,1.15198349698667,-2.38856955364628E-6));
#17822=CARTESIAN_POINT('Ctrl Pts',(10.7951843826221,1.16946861094468,-3.77014304120448E-6));
#17823=CARTESIAN_POINT('Ctrl Pts',(10.7919669771209,1.18718176881198,-5.16973525142236E-6));
#17824=CARTESIAN_POINT('Ctrl Pts',(10.7871724978816,1.20460918321158,-5.4755482503851E-6));
#17825=CARTESIAN_POINT('Ctrl Pts',(10.7808573412527,1.22152732075962,-4.27334038376583E-6));
#17826=CARTESIAN_POINT('Ctrl Pts',(10.7797421066656,1.22451500471617,-4.06103467663179E-6));
#17827=CARTESIAN_POINT('Ctrl Pts',(10.7785793293545,1.22748675045939,-3.81081650224554E-6));
#17828=CARTESIAN_POINT('Ctrl Pts',(10.7773691713543,1.23044124224994,-3.53261416912234E-6));
#17829=CARTESIAN_POINT('Ctrl Pts',(10.7705159051166,1.24717287467681,-1.95712183132163E-6));
#17830=CARTESIAN_POINT('Ctrl Pts',(10.7622076549587,1.26320448426569,8.50150473021234E-7));
#17831=CARTESIAN_POINT('Ctrl Pts',(10.7525236566209,1.27832128496499,1.09915986206012E-6));
#17832=CARTESIAN_POINT('Ctrl Pts',(10.7482509716548,1.28499098118248,1.20902550183604E-6));
#17833=CARTESIAN_POINT('Ctrl Pts',(10.7437098328292,1.29148238441373,7.76315258636623E-7));
#17834=CARTESIAN_POINT('Ctrl Pts',(10.7389041877712,1.29777551763099,-7.54184826032082E-7));
#17835=CARTESIAN_POINT('Ctrl Pts',(10.7310976851069,1.30799836193882,-3.24039694621926E-6));
#17836=CARTESIAN_POINT('Ctrl Pts',(10.7225935645301,1.31769858917671,-8.57388820182801E-6));
#17837=CARTESIAN_POINT('Ctrl Pts',(10.7134588931078,1.3268364513864,-1.41086939541967E-5));
#17838=CARTESIAN_POINT('Ctrl Pts',(10.7004433550849,1.33985653580309,-2.19949628070403E-5));
#17839=CARTESIAN_POINT('Ctrl Pts',(10.6862650266646,1.35162127070648,-3.0022236679635E-5));
#17840=CARTESIAN_POINT('Ctrl Pts',(10.6711476119081,1.36204513612776,-3.40981369893719E-5));
#17841=CARTESIAN_POINT('Ctrl Pts',(10.6560301971515,1.37246900154903,-3.81740372991087E-5));
#17842=CARTESIAN_POINT('Ctrl Pts',(10.6399721826852,1.38155285075117,-3.83332859284948E-5));
#17843=CARTESIAN_POINT('Ctrl Pts',(10.6231652498763,1.38916602817047,-3.45204725343976E-5));
#17844=CARTESIAN_POINT('Ctrl Pts',(10.6063487480974,1.39678354012646,-3.07054883279539E-5));
#17845=CARTESIAN_POINT('Ctrl Pts',(10.5889271210941,1.40286310406803,-2.29928881382306E-5));
#17846=CARTESIAN_POINT('Ctrl Pts',(10.5711041279812,1.40730078588308,-1.53078138731408E-5));
#17847=CARTESIAN_POINT('Ctrl Pts',(10.5532811348684,1.41173846769814,-7.6227396080509E-6));
#17848=CARTESIAN_POINT('Ctrl Pts',(10.5350552605908,1.41453511891929,-9.16729947674095E-11));
#17849=CARTESIAN_POINT('Ctrl Pts',(10.5166159648474,1.4155315881283,2.48932818802672E-16));
#17850=CARTESIAN_POINT('',(10.8,-1.11638029377732,-1.39157997946485E-17));
#17851=CARTESIAN_POINT('',(10.8,1.4,0.));
#17852=CARTESIAN_POINT('',(10.5166159648474,-1.4155315881283,2.77555756156289E-17));
#17853=CARTESIAN_POINT('Ctrl Pts',(10.5166159648474,-1.4155315881283,-1.94289029309402E-16));
#17854=CARTESIAN_POINT('Ctrl Pts',(10.5344251606169,-1.41456917089032,1.72780596414851E-12));
#17855=CARTESIAN_POINT('Ctrl Pts',(10.5520727686739,-1.41197333457428,-2.53403886306205E-6));
#17856=CARTESIAN_POINT('Ctrl Pts',(10.5693578805681,-1.40785843881911,-4.04156906196095E-6));
#17857=CARTESIAN_POINT('Ctrl Pts',(10.5868701251756,-1.40368947182374,-5.56890876087065E-6));
#17858=CARTESIAN_POINT('Ctrl Pts',(10.604011804524,-1.39796079212135,-5.98742339745246E-6));
#17859=CARTESIAN_POINT('Ctrl Pts',(10.6205627760847,-1.39074087128671,-4.81856832951796E-6));
#17860=CARTESIAN_POINT('Ctrl Pts',(10.6234754753687,-1.38947028374636,-4.61286902618664E-6));
#17861=CARTESIAN_POINT('Ctrl Pts',(10.6263698187278,-1.38815339768352,-4.36721670635639E-6));
#17862=CARTESIAN_POINT('Ctrl Pts',(10.629244514885,-1.38679044403738,-4.09122931699412E-6));
#17863=CARTESIAN_POINT('Ctrl Pts',(10.6455827855986,-1.37904412775797,-2.5226612199239E-6));
#17864=CARTESIAN_POINT('Ctrl Pts',(10.6611432679573,-1.36988219838444,3.58605122725343E-7));
#17865=CARTESIAN_POINT('Ctrl Pts',(10.6757157985124,-1.35939560704671,7.40589063327193E-7));
#17866=CARTESIAN_POINT('Ctrl Pts',(10.6821516119741,-1.35476430808026,9.09288478831296E-7));
#17867=CARTESIAN_POINT('Ctrl Pts',(10.6883944859408,-1.34987400891586,5.44816430868337E-7));
#17868=CARTESIAN_POINT('Ctrl Pts',(10.6944246343503,-1.34472976213865,-9.14752338109426E-7));
#17869=CARTESIAN_POINT('Ctrl Pts',(10.7041966733629,-1.33639335368171,-3.28002794718031E-6));
#17870=CARTESIAN_POINT('Ctrl Pts',(10.7134106653983,-1.3273903805878,-8.47259327327479E-6));
#17871=CARTESIAN_POINT('Ctrl Pts',(10.7220307555455,-1.31778973409553,-1.38734771921913E-5));
#17872=CARTESIAN_POINT('Ctrl Pts',(10.7343338492722,-1.3040871333553,-2.15819326638919E-5));
#17873=CARTESIAN_POINT('Ctrl Pts',(10.7453199276401,-1.28929041974124,-2.94555326738194E-5));
#17874=CARTESIAN_POINT('Ctrl Pts',(10.7549158277293,-1.27362793268665,-3.3443536645081E-5));
#17875=CARTESIAN_POINT('Ctrl Pts',(10.7645117278185,-1.25796544563206,-3.74315406163426E-5));
#17876=CARTESIAN_POINT('Ctrl Pts',(10.7727182208071,-1.24143562566754,-3.75750290962259E-5));
#17877=CARTESIAN_POINT('Ctrl Pts',(10.7794153247677,-1.22423716044977,-3.38265125308188E-5));
#17878=CARTESIAN_POINT('Ctrl Pts',(10.7861166764432,-1.20702778690835,-3.00756184258222E-5));
#17879=CARTESIAN_POINT('Ctrl Pts',(10.7912490477072,-1.18929683429644,-2.25107044755726E-5));
#17880=CARTESIAN_POINT('Ctrl Pts',(10.7947196858669,-1.17125359626911,-1.49815203503087E-5));
#17881=CARTESIAN_POINT('Ctrl Pts',(10.7981903240266,-1.15321035824179,-7.45233622504479E-6));
#17882=CARTESIAN_POINT('Ctrl Pts',(10.7999999985278,-1.13485327409571,-1.17780195603766E-10));
#17883=CARTESIAN_POINT('Ctrl Pts',(10.8,-1.11638029377732,-1.38777878078145E-17));
#17884=CARTESIAN_POINT('',(0.276326924564679,-1.42224670711126,-5.55111512312578E-17));
#17885=CARTESIAN_POINT('Ctrl Pts',(10.5166159648474,-1.4155315881283,0.));
#17886=CARTESIAN_POINT('Ctrl Pts',(7.10318628475318,-1.599994843061,0.));
#17887=CARTESIAN_POINT('Ctrl Pts',(3.68975660465893,-1.68747752195839,0.));
#17888=CARTESIAN_POINT('Ctrl Pts',(0.276326924564679,-1.42224670711126,
0.));
#17889=CARTESIAN_POINT('',(-7.25311916552711E-19,-1.12356026268968,1.39157997946485E-17));
#17890=CARTESIAN_POINT('Ctrl Pts',(1.80411241501588E-16,-1.12356026268968,
-1.53523027623947E-16));
#17891=CARTESIAN_POINT('Ctrl Pts',(7.41078168374529E-10,-1.14141522098415,
-1.3067981184062E-11));
#17892=CARTESIAN_POINT('Ctrl Pts',(0.00163694718329378,-1.15920272117896,
-1.78823819589733E-6));
#17893=CARTESIAN_POINT('Ctrl Pts',(0.00481087395297265,-1.17671209893291,
-2.3181425555783E-6));
#17894=CARTESIAN_POINT('Ctrl Pts',(0.00802138847203439,-1.19442331774104,
-2.85415543927884E-6));
#17895=CARTESIAN_POINT('Ctrl Pts',(0.0128049030182357,-1.21185152247087,
-2.04128886843626E-6));
#17896=CARTESIAN_POINT('Ctrl Pts',(0.0191087770915565,-1.22877027194193,
1.71240493184593E-7));
#17897=CARTESIAN_POINT('Ctrl Pts',(0.0202201941454154,-1.23175316571065,
5.613248819379E-7));
#17898=CARTESIAN_POINT('Ctrl Pts',(0.0213789882593307,-1.23472016785247,
9.85829603970989E-7));
#17899=CARTESIAN_POINT('Ctrl Pts',(0.0225850188675993,-1.23766995297306,
1.43287414332239E-6));
#17900=CARTESIAN_POINT('Ctrl Pts',(0.0294291562303479,-1.25440977235863,
3.96981990042924E-6));
#17901=CARTESIAN_POINT('Ctrl Pts',(0.0377300686697735,-1.27044838970616,
7.55798501181421E-6));
#17902=CARTESIAN_POINT('Ctrl Pts',(0.0474121614036163,-1.28556782977674,
8.05058320302158E-6));
#17903=CARTESIAN_POINT('Ctrl Pts',(0.0511425121829324,-1.29139310088294,
8.24037316857697E-6));
#17904=CARTESIAN_POINT('Ctrl Pts',(0.0550784035723718,-1.29708174651376,
7.93435480917585E-6));
#17905=CARTESIAN_POINT('Ctrl Pts',(0.0592173503759339,-1.30262033374061,
6.74858081742264E-6));
#17906=CARTESIAN_POINT('Ctrl Pts',(0.0675201807396794,-1.31373087764993,
4.36988865960166E-6));
#17907=CARTESIAN_POINT('Ctrl Pts',(0.0766394565597649,-1.32423847988766,
-1.46587651676554E-6));
#17908=CARTESIAN_POINT('Ctrl Pts',(0.0864911062490747,-1.33409287340636,
-7.46705500292641E-6));
#17909=CARTESIAN_POINT('Ctrl Pts',(0.0992988409846585,-1.34690417528452,
-1.52689465211603E-5));
#17910=CARTESIAN_POINT('Ctrl Pts',(0.113232871116931,-1.35850278376499,
-2.31308069859054E-5));
#17911=CARTESIAN_POINT('Ctrl Pts',(0.128081622025101,-1.36880445085772,
-2.72849174168177E-5));
#17912=CARTESIAN_POINT('Ctrl Pts',(0.142447925282442,-1.37877140864598,
-3.13040575171566E-5));
#17913=CARTESIAN_POINT('Ctrl Pts',(0.157671864768995,-1.38752483454192,
-3.1899138628041E-5));
#17914=CARTESIAN_POINT('Ctrl Pts',(0.173588691395025,-1.39495074934422,
-2.90326641197332E-5));
#17915=CARTESIAN_POINT('Ctrl Pts',(0.189936400238013,-1.40257769006131,
-2.60885916756054E-5));
#17916=CARTESIAN_POINT('Ctrl Pts',(0.206881864105471,-1.40874232120582,
-1.95409011442111E-5));
#17917=CARTESIAN_POINT('Ctrl Pts',(0.22423558959196,-1.41334558507228,-1.29462590315495E-5));
#17918=CARTESIAN_POINT('Ctrl Pts',(0.241260467995769,-1.4178616186841,-6.47658310103417E-6));
#17919=CARTESIAN_POINT('Ctrl Pts',(0.258679581942429,-1.42087546890512,
-1.12101563992788E-10));
#17920=CARTESIAN_POINT('Ctrl Pts',(0.27632692456468,-1.42224670711126,1.05818132034585E-16));
#17921=CARTESIAN_POINT('',(0.,-1.4,0.));
#17922=CARTESIAN_POINT('',(0.292382661757373,-1.22257596919059,0.));
#17923=CARTESIAN_POINT('Ctrl Pts',(0.200274469199584,-1.12301388185427,
-2.68882138776405E-17));
#17924=CARTESIAN_POINT('Ctrl Pts',(0.200274469314753,-1.13095194822878,
-2.85686379674833E-12));
#17925=CARTESIAN_POINT('Ctrl Pts',(0.201244085522878,-1.13884856843413,
-1.08105759021766E-6));
#17926=CARTESIAN_POINT('Ctrl Pts',(0.203110344361254,-1.14653799330522,
-1.10782444979703E-6));
#17927=CARTESIAN_POINT('Ctrl Pts',(0.204308287281872,-1.15147379958167,
-1.12500597321754E-6));
#17928=CARTESIAN_POINT('Ctrl Pts',(0.205876831658669,-1.15632444796435,
-7.573778542164E-7));
#17929=CARTESIAN_POINT('Ctrl Pts',(0.207807574899602,-1.16104329283393,
-1.57887042599725E-7));
#17930=CARTESIAN_POINT('Ctrl Pts',(0.21096922807971,-1.1687705506961,8.23798139982571E-7));
#17931=CARTESIAN_POINT('Ctrl Pts',(0.215060220496011,-1.17605061753432,
2.67511715935828E-6));
#17932=CARTESIAN_POINT('Ctrl Pts',(0.220020901709485,-1.18268777995331,
1.20301732358232E-6));
#17933=CARTESIAN_POINT('Ctrl Pts',(0.222788929945646,-1.18639127392786,
3.81595076007225E-7));
#17934=CARTESIAN_POINT('Ctrl Pts',(0.225828882930032,-1.18989419630164,
-1.55522758636672E-6));
#17935=CARTESIAN_POINT('Ctrl Pts',(0.229112809647272,-1.19317965616817,
-3.52099818518546E-6));
#17936=CARTESIAN_POINT('Ctrl Pts',(0.234731790749985,-1.1988012605745,-6.88454091865859E-6));
#17937=CARTESIAN_POINT('Ctrl Pts',(0.240999377733319,-1.20372479786492,
-1.00686973618824E-5));
#17938=CARTESIAN_POINT('Ctrl Pts',(0.247759525934523,-1.2078808899968,-1.07387199666626E-5));
#17939=CARTESIAN_POINT('Ctrl Pts',(0.251104201987095,-1.20993717358883,
-1.10702228411842E-5));
#17940=CARTESIAN_POINT('Ctrl Pts',(0.254570062984725,-1.21180502729412,
-1.08478245319173E-5));
#17941=CARTESIAN_POINT('Ctrl Pts',(0.258140701417296,-1.21347208138814,
-1.01264154182862E-5));
#17942=CARTESIAN_POINT('Ctrl Pts',(0.265309933881728,-1.21681924144269,
-8.67794906268977E-6));
#17943=CARTESIAN_POINT('Ctrl Pts',(0.27282354441991,-1.21932394229889,-5.03816435877804E-6));
#17944=CARTESIAN_POINT('Ctrl Pts',(0.280540402387729,-1.22090470300999,
-2.38011023443526E-6));
#17945=CARTESIAN_POINT('Ctrl Pts',(0.284441227387562,-1.22170376798259,
-1.03647996128718E-6));
#17946=CARTESIAN_POINT('Ctrl Pts',(0.288394358015454,-1.22226603782358,
-8.41267709508591E-12));
#17947=CARTESIAN_POINT('Ctrl Pts',(0.292382661757373,-1.22257596919059,
3.10081821330854E-17));
#17948=CARTESIAN_POINT('',(0.9,-1.266106713614,0.));
#17949=CARTESIAN_POINT('Ctrl Pts',(0.29238266175737,-1.22257596919059,3.4274341177698E-16));
#17950=CARTESIAN_POINT('Ctrl Pts',(0.494894519961671,-1.23831317320793,
3.6654050078524E-12));
#17951=CARTESIAN_POINT('Ctrl Pts',(0.697432753591781,-1.25280566766171,
-2.10377631034678E-8));
#17952=CARTESIAN_POINT('Ctrl Pts',(0.900000000000002,-1.266106713614,4.80511808774455E-17));
#17953=CARTESIAN_POINT('',(0.9,1.34328341716202,0.));
#17954=CARTESIAN_POINT('',(3.5,-1.37552980833516,0.));
#17955=CARTESIAN_POINT('Ctrl Pts',(1.10000000028363,-1.27885335028943,-5.13283219638443E-11));
#17956=CARTESIAN_POINT('Ctrl Pts',(1.8994825293422,-1.32827224294784,2.51289069808066E-7));
#17957=CARTESIAN_POINT('Ctrl Pts',(2.69943073922525,-1.35940904940056,2.35357980118634E-7));
#17958=CARTESIAN_POINT('Ctrl Pts',(3.50000000097418,-1.37552980835478,8.59034485311056E-16));
#17959=CARTESIAN_POINT('',(3.5,1.44777777777778,0.));
#17960=CARTESIAN_POINT('',(7.1,-1.35793097395724,0.));
#17961=CARTESIAN_POINT('Ctrl Pts',(3.700000000362,-1.379246395385,-6.25385501848083E-12));
#17962=CARTESIAN_POINT('Ctrl Pts',(4.26467016042339,-1.38886773733237,1.63880713394601E-8));
#17963=CARTESIAN_POINT('Ctrl Pts',(4.82965558050887,-1.39115503781354,-4.12727732537403E-8));
#17964=CARTESIAN_POINT('Ctrl Pts',(5.39500817395676,-1.38725486475042,-3.97626883737645E-8));
#17965=CARTESIAN_POINT('Ctrl Pts',(5.96336684492344,-1.38333395379258,-3.82445741104923E-8));
#17966=CARTESIAN_POINT('Ctrl Pts',(6.53173538886785,-1.37316170188981,3.71969681223073E-9));
#17967=CARTESIAN_POINT('Ctrl Pts',(7.1000000000396,-1.35793097389613,-4.88946831112289E-12));
#17968=CARTESIAN_POINT('',(7.1,1.42555555555556,0.));
#17969=CARTESIAN_POINT('',(10.2,-1.23178301601145,0.));
#17970=CARTESIAN_POINT('',(10.5052647440597,-1.21555035534119,0.));
#17971=CARTESIAN_POINT('Ctrl Pts',(10.2,-1.23178301601145,-4.56855690431079E-17));
#17972=CARTESIAN_POINT('Ctrl Pts',(10.3017652114452,-1.22646242153193,-6.28718440835499E-11));
#17973=CARTESIAN_POINT('Ctrl Pts',(10.4035203469111,-1.22104923788321,1.43982679105611E-13));
#17974=CARTESIAN_POINT('Ctrl Pts',(10.5052647440597,-1.21555035534119,6.44897004721534E-17));
#17975=CARTESIAN_POINT('',(10.5997255308004,-1.11583328740478,1.38777878078145E-17));
#17976=CARTESIAN_POINT('Ctrl Pts',(10.5052647440597,-1.21555035534119,-1.86482773667507E-17));
#17977=CARTESIAN_POINT('Ctrl Pts',(10.5131888530666,-1.21512208850275,-5.60416335832109E-13));
#17978=CARTESIAN_POINT('Ctrl Pts',(10.5210180054001,-1.21372544600509,-1.35972994235015E-6));
#17979=CARTESIAN_POINT('Ctrl Pts',(10.5285917824072,-1.2114444991589,-1.66070161277884E-6));
#17980=CARTESIAN_POINT('Ctrl Pts',(10.5334522234388,-1.20998071066451,-1.8538489757029E-6));
#17981=CARTESIAN_POINT('Ctrl Pts',(10.538207639053,-1.20815156029678,-1.66445033219183E-6));
#17982=CARTESIAN_POINT('Ctrl Pts',(10.542812250732,-1.20596855068549,-1.19054254011085E-6));
#17983=CARTESIAN_POINT('Ctrl Pts',(10.5499808226381,-1.20256998801374,-4.52751316616249E-7));
#17984=CARTESIAN_POINT('Ctrl Pts',(10.5567010840309,-1.19835579238971,1.16775294480959E-6));
#17985=CARTESIAN_POINT('Ctrl Pts',(10.5628099082467,-1.1933896765605,3.12218506849373E-7));
#17986=CARTESIAN_POINT('Ctrl Pts',(10.563392699667,-1.1929159013142,2.30599178383296E-7));
#17987=CARTESIAN_POINT('Ctrl Pts',(10.563969906567,-1.19243524850296,1.23643260424227E-7));
#17988=CARTESIAN_POINT('Ctrl Pts',(10.5645413730323,-1.19194775268147,-1.33988689923433E-8));
#17989=CARTESIAN_POINT('Ctrl Pts',(10.5677990734116,-1.18916873515523,-7.94620907596477E-7));
#17990=CARTESIAN_POINT('Ctrl Pts',(10.5708705204042,-1.18616755700159,-2.52696578471864E-6));
#17991=CARTESIAN_POINT('Ctrl Pts',(10.5737438185805,-1.18296717200411,-4.3349897000341E-6));
#17992=CARTESIAN_POINT('Ctrl Pts',(10.579054042416,-1.17705244973962,-7.67644996655303E-6));
#17993=CARTESIAN_POINT('Ctrl Pts',(10.5836289246435,-1.17052745137283,-1.0999028846932E-5));
#17994=CARTESIAN_POINT('Ctrl Pts',(10.5874112735695,-1.16355342251842,-1.18035167459916E-5));
#17995=CARTESIAN_POINT('Ctrl Pts',(10.5894705469099,-1.15975646143,-1.22415145393192E-5));
#17996=CARTESIAN_POINT('Ctrl Pts',(10.5912942421259,-1.15582570378367,-1.20038889321768E-5));
#17997=CARTESIAN_POINT('Ctrl Pts',(10.5928674986933,-1.15178403025788,-1.11465830745351E-5));
#17998=CARTESIAN_POINT('Ctrl Pts',(10.5957384082276,-1.14440870489779,-9.58215448007377E-6));
#17999=CARTESIAN_POINT('Ctrl Pts',(10.5977463817932,-1.13674651935037,-5.80208140981121E-6));
#18000=CARTESIAN_POINT('Ctrl Pts',(10.5988207707371,-1.12894377506163,-2.8960211281105E-6));
#18001=CARTESIAN_POINT('Ctrl Pts',(10.5994175893465,-1.12460938291963,-1.28171667533415E-6));
#18002=CARTESIAN_POINT('Ctrl Pts',(10.5997255306822,-1.12023121224821,-9.4020583932734E-12));
#18003=CARTESIAN_POINT('Ctrl Pts',(10.5997255308004,-1.11583328740478,-9.97465998686664E-18));
#18004=CARTESIAN_POINT('',(10.5997255308004,1.11583328740478,0.));
#18005=CARTESIAN_POINT('',(10.5997255308004,0.7,0.));
#18006=CARTESIAN_POINT('',(10.5052647440597,1.21555035534119,0.));
#18007=CARTESIAN_POINT('Ctrl Pts',(10.5997255308004,1.11583328740478,8.8037216405823E-17));
#18008=CARTESIAN_POINT('Ctrl Pts',(10.5997255307124,1.12376989384288,-2.22024716398596E-12));
#18009=CARTESIAN_POINT('Ctrl Pts',(10.5987536115518,1.13166401228391,-1.27532141444775E-6));
#18010=CARTESIAN_POINT('Ctrl Pts',(10.5968849989732,1.13935090273995,-1.5236651967046E-6));
#18011=CARTESIAN_POINT('Ctrl Pts',(10.5956849616024,1.14428748291596,-1.68315348385219E-6));
#18012=CARTESIAN_POINT('Ctrl Pts',(10.5941139374364,1.14913880701507,-1.46899737395989E-6));
#18013=CARTESIAN_POINT('Ctrl Pts',(10.5921809408638,1.1538584293407,-9.90118991603547E-7));
#18014=CARTESIAN_POINT('Ctrl Pts',(10.5891742477341,1.16119959911942,-2.45244239835432E-7));
#18015=CARTESIAN_POINT('Ctrl Pts',(10.5853292249979,1.16813727090899,1.33309554558619E-6));
#18016=CARTESIAN_POINT('Ctrl Pts',(10.5807005079991,1.17450509276749,4.08358240744415E-7));
#18017=CARTESIAN_POINT('Ctrl Pts',(10.5802604812716,1.17511044665166,3.20448539159982E-7));
#18018=CARTESIAN_POINT('Ctrl Pts',(10.5798133373602,1.17571063303672,2.07176952714776E-7));
#18019=CARTESIAN_POINT('Ctrl Pts',(10.5793591019426,1.17630549598644,6.38823567561716E-8));
#18020=CARTESIAN_POINT('Ctrl Pts',(10.5767566952267,1.17971358631841,-7.57081408668461E-7));
#18021=CARTESIAN_POINT('Ctrl Pts',(10.5739217504488,1.18294722379721,-2.53660858190298E-6));
#18022=CARTESIAN_POINT('Ctrl Pts',(10.570876618072,1.18599321478588,-4.38998728286835E-6));
#18023=CARTESIAN_POINT('Ctrl Pts',(10.5652565693637,1.19161484813492,-7.81055403847458E-6));
#18024=CARTESIAN_POINT('Ctrl Pts',(10.5589874561388,1.19653507038546,-1.11999964534866E-5));
#18025=CARTESIAN_POINT('Ctrl Pts',(10.5522271124844,1.20068789486255,-1.20263298844839E-5));
#18026=CARTESIAN_POINT('Ctrl Pts',(10.5485500617744,1.20294667739977,-1.24757848359648E-5));
#18027=CARTESIAN_POINT('Ctrl Pts',(10.5447269560479,1.20497781184918,-1.22374322375965E-5));
#18028=CARTESIAN_POINT('Ctrl Pts',(10.5407797717187,1.20676523914267,-1.13674773191707E-5));
#18029=CARTESIAN_POINT('Ctrl Pts',(10.5335711832013,1.210029547771,-9.77871264224002E-6));
#18030=CARTESIAN_POINT('Ctrl Pts',(10.5260296312848,1.21244761587922,-5.9245235663186E-6));
#18031=CARTESIAN_POINT('Ctrl Pts',(10.5182973307397,1.21394093281975,-2.95733858081469E-6));
#18032=CARTESIAN_POINT('Ctrl Pts',(10.514004731837,1.21476995008607,-1.31010113336685E-6));
#18033=CARTESIAN_POINT('Ctrl Pts',(10.5096528988527,1.21531319279956,-7.28166367327128E-12));
#18034=CARTESIAN_POINT('Ctrl Pts',(10.5052647440597,1.21555035534119,-3.31765864780564E-17));
#18035=CARTESIAN_POINT('',(10.2,1.23178301601145,0.));
#18036=CARTESIAN_POINT('Ctrl Pts',(10.5052647440597,1.21555035534119,1.20285454773689E-16));
#18037=CARTESIAN_POINT('Ctrl Pts',(10.4035203468995,1.22104923788384,1.44021921739714E-13));
#18038=CARTESIAN_POINT('Ctrl Pts',(10.3017652114309,1.22646242153268,-6.28696045710378E-11));
#18039=CARTESIAN_POINT('Ctrl Pts',(10.2,1.23178301601145,1.23125603768043E-16));
#18040=CARTESIAN_POINT('',(10.2,-1.30754691548544,0.));
#18041=CARTESIAN_POINT('Origin',(8.8,0.,0.));
#18042=CARTESIAN_POINT('',(8.4,-4.89858719658942E-17,0.));
#18043=CARTESIAN_POINT('Origin',(2.,0.,0.));
#18044=CARTESIAN_POINT('',(1.6,-4.89858719658941E-17,0.7));
#18045=CARTESIAN_POINT('Origin',(2.,0.,0.7));
#18046=CARTESIAN_POINT('',(1.6,-4.89858719658941E-17,0.));
#18047=CARTESIAN_POINT('Origin',(10.2,-1.30754691548544,0.));
#18048=CARTESIAN_POINT('',(10.1999999975107,-1.19856231453552,0.605472757505173));
#18049=CARTESIAN_POINT('Ctrl Pts',(10.2,-1.23178301601145,0.));
#18050=CARTESIAN_POINT('Ctrl Pts',(10.2,-1.22625045235593,0.100869147801815));
#18051=CARTESIAN_POINT('Ctrl Pts',(10.2,-1.22071692450357,0.201739022585575));
#18052=CARTESIAN_POINT('Ctrl Pts',(10.2,-1.2096433936729,0.403562754186249));
#18053=CARTESIAN_POINT('Ctrl Pts',(10.1999999975107,-1.20410330368611,0.50451817268257));
#18054=CARTESIAN_POINT('Ctrl Pts',(10.1999999975107,-1.19856231453552,0.605472757505173));
#18055=CARTESIAN_POINT('',(10.1999999975107,1.19856231453552,0.605472757505173));
#18056=CARTESIAN_POINT('Ctrl Pts',(10.1999999975107,1.19856231453552,0.605472757505173));
#18057=CARTESIAN_POINT('Ctrl Pts',(10.1999999975107,1.20410418062036,0.504502195294633));
#18058=CARTESIAN_POINT('Ctrl Pts',(10.2,1.20964514726505,0.403530798997214));
#18059=CARTESIAN_POINT('Ctrl Pts',(10.2,1.22071867750565,0.201707067365009));
#18060=CARTESIAN_POINT('Ctrl Pts',(10.2,1.22625132869937,0.100853170395858));
#18061=CARTESIAN_POINT('Ctrl Pts',(10.2,1.23178301601145,0.));
#18062=CARTESIAN_POINT('',(10.1999999980542,1.09857320530976,0.7));
#18063=CARTESIAN_POINT('Ctrl Pts',(10.1999999999973,1.09857320510493,0.7));
#18064=CARTESIAN_POINT('Ctrl Pts',(10.2000000008642,1.10649088744708,0.699999999248278));
#18065=CARTESIAN_POINT('Ctrl Pts',(10.1999989363772,1.11434529358656,0.699006164779054));
#18066=CARTESIAN_POINT('Ctrl Pts',(10.1999980093114,1.12199598895487,0.697118997523365));
#18067=CARTESIAN_POINT('Ctrl Pts',(10.1999974900707,1.12628106973794,0.696062013320951));
#18068=CARTESIAN_POINT('Ctrl Pts',(10.1999970168623,1.13050229860485,0.694723760583242));
#18069=CARTESIAN_POINT('Ctrl Pts',(10.199996713894,1.13463332887353,0.693115046692397));
#18070=CARTESIAN_POINT('Ctrl Pts',(10.1999961690675,1.14206214329588,0.690222103243312));
#18071=CARTESIAN_POINT('Ctrl Pts',(10.1999962772589,1.14911941279843,0.686488866209959));
#18072=CARTESIAN_POINT('Ctrl Pts',(10.1999969599022,1.15565885618684,0.681996408643444));
#18073=CARTESIAN_POINT('Ctrl Pts',(10.1999973343062,1.15924549304116,0.679532465931891));
#18074=CARTESIAN_POINT('Ctrl Pts',(10.1999978674396,1.16267609380848,0.676839263748528));
#18075=CARTESIAN_POINT('Ctrl Pts',(10.1999983417863,1.16592263776853,0.673924718551186));
#18076=CARTESIAN_POINT('Ctrl Pts',(10.199998806773,1.16910511991263,0.671067684066867));
#18077=CARTESIAN_POINT('Ctrl Pts',(10.1999992207276,1.17209141256199,0.668015240668471));
#18078=CARTESIAN_POINT('Ctrl Pts',(10.1999992206607,1.17485880184773,0.664778864469812));
#18079=CARTESIAN_POINT('Ctrl Pts',(10.1999992205369,1.17997899231675,0.658790960038769));
#18080=CARTESIAN_POINT('Ctrl Pts',(10.1999979581638,1.18435276586188,0.652174799271591));
#18081=CARTESIAN_POINT('Ctrl Pts',(10.1999975326045,1.18791964688485,0.645095405674036));
#18082=CARTESIAN_POINT('Ctrl Pts',(10.1999974898604,1.18827791229431,0.644384335742179));
#18083=CARTESIAN_POINT('Ctrl Pts',(10.1999974535047,1.18862799840101,0.643668573506599));
#18084=CARTESIAN_POINT('Ctrl Pts',(10.1999974242393,1.18896981696374,0.64294827577739));
#18085=CARTESIAN_POINT('Ctrl Pts',(10.1999971329942,1.1923715530028,0.635779961907205));
#18086=CARTESIAN_POINT('Ctrl Pts',(10.1999977790614,1.19491900203126,0.628247233077589));
#18087=CARTESIAN_POINT('Ctrl Pts',(10.1999987199397,1.19655829940385,0.620518158911201));
#18088=CARTESIAN_POINT('Ctrl Pts',(10.1999993222661,1.19760773597399,0.615570201805241));
#18089=CARTESIAN_POINT('Ctrl Pts',(10.2,1.19828413277105,0.610541112135461));
#18090=CARTESIAN_POINT('Ctrl Pts',(10.2,1.19856231427281,0.60547275750556));
#18091=CARTESIAN_POINT('',(10.2,-1.09857320510402,0.7));
#18092=CARTESIAN_POINT('',(10.2,-0.653773457742722,0.7));
#18093=CARTESIAN_POINT('Ctrl Pts',(10.2,-1.19856231427281,0.60547275750556));
#18094=CARTESIAN_POINT('Ctrl Pts',(10.2,-1.19812809376428,0.613384079828744));
#18095=CARTESIAN_POINT('Ctrl Pts',(10.1999984889428,-1.1967261327477,0.621202329970501));
#18096=CARTESIAN_POINT('Ctrl Pts',(10.1999978161146,-1.19444079525024,0.628767398200536));
#18097=CARTESIAN_POINT('Ctrl Pts',(10.1999974438306,-1.19317629038787,0.632953241898348));
#18098=CARTESIAN_POINT('Ctrl Pts',(10.1999972759003,-1.19164034846853,0.637061602680377));
#18099=CARTESIAN_POINT('Ctrl Pts',(10.1999973648938,-1.18984073583679,0.641063423920242));
#18100=CARTESIAN_POINT('Ctrl Pts',(10.1999975257516,-1.18658789218766,0.648296813248274));
#18101=CARTESIAN_POINT('Ctrl Pts',(10.1999986492083,-1.18251199594868,0.655103972585077));
#18102=CARTESIAN_POINT('Ctrl Pts',(10.1999990866637,-1.1776776067306,0.66132208754656));
#18103=CARTESIAN_POINT('Ctrl Pts',(10.1999991692372,-1.17676507450965,0.662495809810115));
#18104=CARTESIAN_POINT('Ctrl Pts',(10.1999992204458,-1.17582538639523,0.663648473741297));
#18105=CARTESIAN_POINT('Ctrl Pts',(10.1999992199672,-1.17485880188435,0.664778864469789));
#18106=CARTESIAN_POINT('Ctrl Pts',(10.1999992190419,-1.17299032792757,0.666963987046661));
#18107=CARTESIAN_POINT('Ctrl Pts',(10.1999990265713,-1.17102137903347,0.669065925022507));
#18108=CARTESIAN_POINT('Ctrl Pts',(10.1999987631451,-1.16895889720817,0.671081139337088));
#18109=CARTESIAN_POINT('Ctrl Pts',(10.1999980371048,-1.16327440276409,0.676635357771578));
#18110=CARTESIAN_POINT('Ctrl Pts',(10.1999968952367,-1.15694629605269,0.681471105251756));
#18111=CARTESIAN_POINT('Ctrl Pts',(10.1999965193249,-1.15013861030111,0.685534582868085));
#18112=CARTESIAN_POINT('Ctrl Pts',(10.1999962798276,-1.14580136285465,0.688123466749966));
#18113=CARTESIAN_POINT('Ctrl Pts',(10.1999963003895,-1.14126848503633,0.690398200126003));
#18114=CARTESIAN_POINT('Ctrl Pts',(10.1999965837416,-1.13657664085124,0.692335536714198));
#18115=CARTESIAN_POINT('Ctrl Pts',(10.199997026059,-1.12925259320479,0.695359751696499));
#18116=CARTESIAN_POINT('Ctrl Pts',(10.1999981114625,-1.12162598460505,0.697529439192009));
#18117=CARTESIAN_POINT('Ctrl Pts',(10.1999989867727,-1.11384404680861,0.698775198878229));
#18118=CARTESIAN_POINT('Ctrl Pts',(10.1999995533653,-1.10880676031141,0.699581585232154));
#18119=CARTESIAN_POINT('Ctrl Pts',(10.200000000559,-1.10370379302489,0.699999999512891));
#18120=CARTESIAN_POINT('Ctrl Pts',(10.1999999999973,-1.09857320510493,0.7));
#18121=CARTESIAN_POINT('Ctrl Pts',(10.0273290644374,-1.24073895154929,-0.000342977371441382));
#18122=CARTESIAN_POINT('Ctrl Pts',(10.0182194939277,-1.2301570933055,0.201590462913323));
#18123=CARTESIAN_POINT('Ctrl Pts',(10.0091098064739,-1.21957524432673,0.403523898419685));
#18124=CARTESIAN_POINT('Ctrl Pts',(10.,-1.20899340483173,0.605457329065658));
#18125=CARTESIAN_POINT('Ctrl Pts',(9.11786336174441,-1.287320026752,-0.000205293215301774));
#18126=CARTESIAN_POINT('Ctrl Pts',(9.11054075262461,-1.27673792859995,0.201728409731728));
#18127=CARTESIAN_POINT('Ctrl Pts',(9.10321803982027,-1.2661558351744,0.403662109352091));
#18128=CARTESIAN_POINT('Ctrl Pts',(9.09589522044064,-1.25557375159922,0.605595805683776));
#18129=CARTESIAN_POINT('Ctrl Pts',(8.20875307681921,-1.32613868191631,-8.19769783003664E-5));
#18130=CARTESIAN_POINT('Ctrl Pts',(8.20321812688803,-1.31555630757271,0.201851960079368));
#18131=CARTESIAN_POINT('Ctrl Pts',(8.19768309032111,-1.30497393555236,0.403785895133155));
#18132=CARTESIAN_POINT('Ctrl Pts',(8.19214796413157,-1.29439157095064,0.605719828258773));
#18133=CARTESIAN_POINT('Ctrl Pts',(7.29999999999999,-1.35236351479115,1.04083408558608E-17));
#18134=CARTESIAN_POINT('Ctrl Pts',(7.29625341766944,-1.34178092325774,0.201934092022114));
#18135=CARTESIAN_POINT('Ctrl Pts',(7.2925067690755,-1.33119833465137,0.403868182971915));
#18136=CARTESIAN_POINT('Ctrl Pts',(7.28876005303739,-1.32061574904145,0.605802272831199));
#18137=CARTESIAN_POINT('Ctrl Pts',(7.29999999953094,-1.32031613471704,0.605285370449856));
#18138=CARTESIAN_POINT('Ctrl Pts',(8.20058408060299,-1.29406305600824,0.605326635812744));
#18139=CARTESIAN_POINT('Ctrl Pts',(9.10058974048747,-1.25534320916473,0.605388449123016));
#18140=CARTESIAN_POINT('Ctrl Pts',(9.99999999968202,-1.20899340489109,0.605457329065633));
#18141=CARTESIAN_POINT('Ctrl Pts',(10.5052670937641,-1.21555282972197,-4.72190879230918E-5));
#18142=CARTESIAN_POINT('Ctrl Pts',(10.4952228315222,-1.20497561405085,0.201799837144789));
#18143=CARTESIAN_POINT('Ctrl Pts',(10.4851784461209,-1.19439840869387,0.403646887802288));
#18144=CARTESIAN_POINT('Ctrl Pts',(10.4751339353761,-1.18382121389426,0.605493932788863));
#18145=CARTESIAN_POINT('Ctrl Pts',(10.4035069533234,-1.22105168617584,-3.13467776074076E-5));
#18146=CARTESIAN_POINT('Ctrl Pts',(10.3936624949941,-1.21047444506522,0.201815739766394));
#18147=CARTESIAN_POINT('Ctrl Pts',(10.3838179147697,-1.19989721405033,0.403662820908308));
#18148=CARTESIAN_POINT('Ctrl Pts',(10.3739732104882,-1.18931999337004,0.605509896555428));
#18149=CARTESIAN_POINT('Ctrl Pts',(10.3017512542637,-1.22646400658821,-1.55943981238903E-5));
#18150=CARTESIAN_POINT('Ctrl Pts',(10.2921066085356,-1.21588673949083,0.201831522212972));
#18151=CARTESIAN_POINT('Ctrl Pts',(10.2824618422276,-1.20530948226626,0.403678633593635));
#18152=CARTESIAN_POINT('Ctrl Pts',(10.2728169532007,-1.19473223514815,0.605525739654126));
#18153=CARTESIAN_POINT('Ctrl Pts',(10.2,-1.23178301601145,-4.5102810375397E-17));
#18154=CARTESIAN_POINT('Ctrl Pts',(10.1905551755811,-1.22120572247414,0.20184714636246));
#18155=CARTESIAN_POINT('Ctrl Pts',(10.1811102319487,-1.21062843858304,0.403694287664275));
#18156=CARTESIAN_POINT('Ctrl Pts',(10.1716651669877,-1.20005116456574,0.605541423818621));
#18157=CARTESIAN_POINT('',(10.4735630903435,-1.18390659316268,0.605494180667944));
#18158=CARTESIAN_POINT('Ctrl Pts',(10.1999999975038,-1.19856231440453,0.605472757505366));
#18159=CARTESIAN_POINT('Ctrl Pts',(10.2911933328565,-1.19375025772558,0.605479840815741));
#18160=CARTESIAN_POINT('Ctrl Pts',(10.3823809652617,-1.18886335120032,0.605486986548286));
#18161=CARTESIAN_POINT('Ctrl Pts',(10.4735630903435,-1.18390659316268,0.605494180667944));
#18162=CARTESIAN_POINT('Ctrl Pts',(10.4735630903435,-1.18390659316268,0.605494180667945));
#18163=CARTESIAN_POINT('Ctrl Pts',(10.4841302498201,-1.19445434834508,0.403662775875149));
#18164=CARTESIAN_POINT('Ctrl Pts',(10.4946974680575,-1.20500226999407,0.201831382381129));
#18165=CARTESIAN_POINT('Ctrl Pts',(10.5052647440597,-1.21555035534119,-6.86299975183324E-17));
#18166=CARTESIAN_POINT('Ctrl Pts',(10.,-1.10900986674273,0.7));
#18167=CARTESIAN_POINT('Ctrl Pts',(9.09944331332257,-1.15544418981837,0.7));
#18168=CARTESIAN_POINT('Ctrl Pts',(8.1984670949788,-1.19422430779862,0.7));
#18169=CARTESIAN_POINT('Ctrl Pts',(7.29709043526679,-1.22049830417059,0.7));
#18170=CARTESIAN_POINT('Ctrl Pts',(10.0014871213396,-1.13785139984992,0.7));
#18171=CARTESIAN_POINT('Ctrl Pts',(9.10076698492608,-1.18430758604571,0.700000491839571));
#18172=CARTESIAN_POINT('Ctrl Pts',(8.19957769811723,-1.22310890030201,0.699999704549177));
#18173=CARTESIAN_POINT('Ctrl Pts',(7.29793284700475,-1.24939875264889,0.7));
#18174=CARTESIAN_POINT('Ctrl Pts',(10.0040646682326,-1.18784086746588,0.676686753673613));
#18175=CARTESIAN_POINT('Ctrl Pts',(9.10306300621911,-1.23433322993607,0.676664155483858));
#18176=CARTESIAN_POINT('Ctrl Pts',(8.20149954052229,-1.27317186922949,0.676644146017133));
#18177=CARTESIAN_POINT('Ctrl Pts',(7.29939288958795,-1.29948813715084,0.676630595533454));
#18178=CARTESIAN_POINT('Ctrl Pts',(10.0050807923581,-1.20754778500352,0.627085325222079));
#18179=CARTESIAN_POINT('Ctrl Pts',(9.10396596140607,-1.25402923300358,0.627026849623412));
#18180=CARTESIAN_POINT('Ctrl Pts',(8.20225661204673,-1.29285896783792,0.626974637782525));
#18181=CARTESIAN_POINT('Ctrl Pts',(7.29996660609514,-1.31917051289423,0.626939603849942));
#18182=CARTESIAN_POINT('Ctrl Pts',(10.0051416645797,-1.20872835322339,0.605457722909465));
#18183=CARTESIAN_POINT('Ctrl Pts',(9.1040197884667,-1.25519559703033,0.605388684776982));
#18184=CARTESIAN_POINT('Ctrl Pts',(8.20230020786566,-1.29401302889245,0.605326714446839));
#18185=CARTESIAN_POINT('Ctrl Pts',(7.29999999953094,-1.32031613471704,0.605285370449856));
#18186=CARTESIAN_POINT('Ctrl Pts',(10.4681436286308,-1.08420482079362,0.7));
#18187=CARTESIAN_POINT('Ctrl Pts',(10.3770124662346,-1.0891584122264,0.7));
#18188=CARTESIAN_POINT('Ctrl Pts',(10.285877616441,-1.09404209584202,0.7));
#18189=CARTESIAN_POINT('Ctrl Pts',(10.1947388861048,-1.09885088260188,0.7));
#18190=CARTESIAN_POINT('Ctrl Pts',(10.4697107510168,-1.11303515260326,0.7));
#18191=CARTESIAN_POINT('Ctrl Pts',(10.3785648662465,-1.11799094453753,0.700000051218742));
#18192=CARTESIAN_POINT('Ctrl Pts',(10.2874149314686,-1.12287675076168,0.699999949550842));
#18193=CARTESIAN_POINT('Ctrl Pts',(10.196260416419,-1.12768774893097,0.7));
#18194=CARTESIAN_POINT('Ctrl Pts',(10.4724269697127,-1.16300539549315,0.676698381019543));
#18195=CARTESIAN_POINT('Ctrl Pts',(10.3812557252598,-1.16796482352885,0.676696026813929));
#18196=CARTESIAN_POINT('Ctrl Pts',(10.2900793016129,-1.17285439035486,0.676693724638983));
#18197=CARTESIAN_POINT('Ctrl Pts',(10.1988975981852,-1.17766904563614,0.67669140632491));
#18198=CARTESIAN_POINT('Ctrl Pts',(10.4734985149421,-1.18271860027509,0.627116141711795));
#18199=CARTESIAN_POINT('Ctrl Pts',(10.382317043787,-1.18767684023183,0.627110048826767));
#18200=CARTESIAN_POINT('Ctrl Pts',(10.2911301919381,-1.19256517083271,0.627104033151799));
#18201=CARTESIAN_POINT('Ctrl Pts',(10.1999375452555,-1.19737868557977,0.627098033786781));
#18202=CARTESIAN_POINT('Ctrl Pts',(10.4735630903435,-1.18390659316268,0.605494180667944));
#18203=CARTESIAN_POINT('Ctrl Pts',(10.3823809652617,-1.18886335120032,0.605486986548286));
#18204=CARTESIAN_POINT('Ctrl Pts',(10.2911933328565,-1.19375025772558,0.605479840815741));
#18205=CARTESIAN_POINT('Ctrl Pts',(10.1999999975038,-1.19856231440453,0.605472757505366));
#18206=CARTESIAN_POINT('',(10.4681436258201,-1.08420482094639,0.7));
#18207=CARTESIAN_POINT('Ctrl Pts',(10.4681436258201,-1.0842048209464,0.7));
#18208=CARTESIAN_POINT('Ctrl Pts',(10.3787660248044,-1.08906309452597,0.7));
#18209=CARTESIAN_POINT('Ctrl Pts',(10.289384876933,-1.09385412476048,0.7));
#18210=CARTESIAN_POINT('Ctrl Pts',(10.1999999999973,-1.09857320510493,0.7));
#18211=CARTESIAN_POINT('Origin',(10.4681436286308,-1.08420482099672,0.6));
#18212=CARTESIAN_POINT('Origin',(5.4,-8.11656130105013E-18,0.7));
#18213=CARTESIAN_POINT('',(10.4681436286308,1.08420482109828,0.7));
#18214=CARTESIAN_POINT('Ctrl Pts',(10.1999999980461,1.09857320520795,0.7));
#18215=CARTESIAN_POINT('Ctrl Pts',(10.2893848765692,1.09385412478074,0.7));
#18216=CARTESIAN_POINT('Ctrl Pts',(10.3787660260279,1.08906309446088,0.7));
#18217=CARTESIAN_POINT('Ctrl Pts',(10.4681436286308,1.08420482079361,0.7));
#18218=CARTESIAN_POINT('',(10.4681436286308,0.7,0.7));
#18219=CARTESIAN_POINT('Ctrl Pts',(7.3,1.35236351479305,-3.57463069561303E-11));
#18220=CARTESIAN_POINT('Ctrl Pts',(7.29625341766908,1.34178092325856,0.20193409200674));
#18221=CARTESIAN_POINT('Ctrl Pts',(7.29250676907475,1.33119833465113,0.403868182976914));
#18222=CARTESIAN_POINT('Ctrl Pts',(7.28876005303626,1.32061574904014,0.60580227285657));
#18223=CARTESIAN_POINT('Ctrl Pts',(8.20875307682014,1.32613868191819,-8.19770140467192E-5));
#18224=CARTESIAN_POINT('Ctrl Pts',(8.20321812688841,1.31555630757352,0.201851960063995));
#18225=CARTESIAN_POINT('Ctrl Pts',(8.19768309032092,1.3049739355521,0.403785895138154));
#18226=CARTESIAN_POINT('Ctrl Pts',(8.19214796413082,1.29439157094932,0.605719828284144));
#18227=CARTESIAN_POINT('Ctrl Pts',(9.11786336174626,1.28732002675385,-0.000205293251048056));
#18228=CARTESIAN_POINT('Ctrl Pts',(9.11054075262572,1.27673792860073,0.201728409716354));
#18229=CARTESIAN_POINT('Ctrl Pts',(9.10321803982063,1.26615583517412,0.403662109357089));
#18230=CARTESIAN_POINT('Ctrl Pts',(9.09589522044026,1.25557375159787,0.605595805709147));
#18231=CARTESIAN_POINT('Ctrl Pts',(10.0273290644402,1.2407389515511,-0.000342977407187712));
#18232=CARTESIAN_POINT('Ctrl Pts',(10.0182194939295,1.23015709330624,0.201590462897949));
#18233=CARTESIAN_POINT('Ctrl Pts',(10.0091098064748,1.21957524432641,0.403523898424684));
#18234=CARTESIAN_POINT('Ctrl Pts',(10.,1.20899340483035,0.605457329091028));
#18235=CARTESIAN_POINT('Ctrl Pts',(10.2,1.23178301601276,-2.39624899783797E-11));
#18236=CARTESIAN_POINT('Ctrl Pts',(10.1905551755807,1.22120572247504,0.201847146346486));
#18237=CARTESIAN_POINT('Ctrl Pts',(10.1811102319479,1.21062843858352,0.403694287656288));
#18238=CARTESIAN_POINT('Ctrl Pts',(10.1716651669865,1.2000511645658,0.605541423818621));
#18239=CARTESIAN_POINT('Ctrl Pts',(10.3017512542641,1.22646400658951,-1.55944220863836E-5));
#18240=CARTESIAN_POINT('Ctrl Pts',(10.2921066085356,1.2158867394917,0.201831522196997));
#18241=CARTESIAN_POINT('Ctrl Pts',(10.2824618422272,1.20530948226672,0.403678633585648));
#18242=CARTESIAN_POINT('Ctrl Pts',(10.2728169531999,1.19473223514819,0.605525739654127));
#18243=CARTESIAN_POINT('Ctrl Pts',(10.4035069533242,1.22105168617711,-3.13468015701665E-5));
#18244=CARTESIAN_POINT('Ctrl Pts',(10.3936624949945,1.21047444506608,0.201815739750419));
#18245=CARTESIAN_POINT('Ctrl Pts',(10.3838179147698,1.19989721405077,0.40366282090032));
#18246=CARTESIAN_POINT('Ctrl Pts',(10.3739732104878,1.18931999337006,0.605509896555428));
#18247=CARTESIAN_POINT('Ctrl Pts',(10.5052670937653,1.21555282972323,-4.72191118859062E-5));
#18248=CARTESIAN_POINT('Ctrl Pts',(10.495222831523,1.20497561405169,0.201799837128814));
#18249=CARTESIAN_POINT('Ctrl Pts',(10.4851784461213,1.19439840869429,0.403646887794301));
#18250=CARTESIAN_POINT('Ctrl Pts',(10.4751339353761,1.18382121389426,0.605493932788864));
#18251=CARTESIAN_POINT('',(10.4735630903435,1.18390659316268,0.605494180667944));
#18252=CARTESIAN_POINT('Ctrl Pts',(10.5052647440597,1.21555035534119,-4.0462425077159E-16));
#18253=CARTESIAN_POINT('Ctrl Pts',(10.4946974680575,1.20500226999407,0.201831382381129));
#18254=CARTESIAN_POINT('Ctrl Pts',(10.4841302498201,1.19445434834508,0.40366277587515));
#18255=CARTESIAN_POINT('Ctrl Pts',(10.4735630903435,1.18390659316268,0.605494180667945));
#18256=CARTESIAN_POINT('Ctrl Pts',(10.4735630903435,1.18390659316268,0.605494180667944));
#18257=CARTESIAN_POINT('Ctrl Pts',(10.3823809652617,1.18886335120032,0.605486986548286));
#18258=CARTESIAN_POINT('Ctrl Pts',(10.2911933328565,1.19375025772558,0.605479840815741));
#18259=CARTESIAN_POINT('Ctrl Pts',(10.1999999975038,1.19856231440453,0.605472757505366));
#18260=CARTESIAN_POINT('Origin',(7.1,1.42555555555556,0.));
#18261=CARTESIAN_POINT('',(7.0999999994629,-1.32593912634735,0.605276549957215));
#18262=CARTESIAN_POINT('Ctrl Pts',(7.0999999994629,-1.32593912634735,0.605276549957215));
#18263=CARTESIAN_POINT('Ctrl Pts',(7.0999999994629,-1.33126650931098,0.504490734647167));
#18264=CARTESIAN_POINT('Ctrl Pts',(7.1,-1.33659376385849,0.403703958452373));
#18265=CARTESIAN_POINT('Ctrl Pts',(7.1,-1.3472576786761,0.201945747207886));
#18266=CARTESIAN_POINT('Ctrl Pts',(7.1,-1.35259443928223,0.100972400854069));
#18267=CARTESIAN_POINT('Ctrl Pts',(7.1,-1.35793097395724,0.));
#18268=CARTESIAN_POINT('',(7.1,-1.22604182196417,0.7));
#18269=CARTESIAN_POINT('Ctrl Pts',(7.1,-1.22604182196307,0.7));
#18270=CARTESIAN_POINT('Ctrl Pts',(7.1,-1.23395163718705,0.7));
#18271=CARTESIAN_POINT('Ctrl Pts',(7.09999945440688,-1.24179783218049,0.699006056038995));
#18272=CARTESIAN_POINT('Ctrl Pts',(7.09999897931553,-1.2494401870438,0.697119011207626));
#18273=CARTESIAN_POINT('Ctrl Pts',(7.09999871186578,-1.25374240366384,0.696056710937424));
#18274=CARTESIAN_POINT('Ctrl Pts',(7.09999846845149,-1.25798007942473,0.69471034534287));
#18275=CARTESIAN_POINT('Ctrl Pts',(7.09999831430822,-1.26212651101681,0.6930909329195));
#18276=CARTESIAN_POINT('Ctrl Pts',(7.09999803835695,-1.26954956016987,0.690191818885951));
#18277=CARTESIAN_POINT('Ctrl Pts',(7.09999810102228,-1.27659977900265,0.686452252582521));
#18278=CARTESIAN_POINT('Ctrl Pts',(7.09999845706054,-1.28313109767173,0.681953977461377));
#18279=CARTESIAN_POINT('Ctrl Pts',(7.09999865314126,-1.2867280867584,0.679476645189077));
#18280=CARTESIAN_POINT('Ctrl Pts',(7.09999893113315,-1.29016742765117,0.67676830886676));
#18281=CARTESIAN_POINT('Ctrl Pts',(7.09999917787259,-1.2934208019838,0.673837071833988));
#18282=CARTESIAN_POINT('Ctrl Pts',(7.09999941835505,-1.29659167515528,0.670980166997299));
#18283=CARTESIAN_POINT('Ctrl Pts',(7.09999963169439,-1.29956664557352,0.667928795646746));
#18284=CARTESIAN_POINT('Ctrl Pts',(7.09999963110542,-1.30232317314677,0.664694459428825));
#18285=CARTESIAN_POINT('Ctrl Pts',(7.09999963001387,-1.30743194453681,0.658700148145236));
#18286=CARTESIAN_POINT('Ctrl Pts',(7.09999897381858,-1.31179333085743,0.652078782729069));
#18287=CARTESIAN_POINT('Ctrl Pts',(7.09999874753952,-1.31534789998199,0.64499600756552));
#18288=CARTESIAN_POINT('Ctrl Pts',(7.09999872438549,-1.31571162172319,0.644271261689237));
#18289=CARTESIAN_POINT('Ctrl Pts',(7.0999987046402,-1.31606685549941,0.643541664816448));
#18290=CARTESIAN_POINT('Ctrl Pts',(7.09999868869212,-1.31641350913238,0.642807383257706));
#18291=CARTESIAN_POINT('Ctrl Pts',(7.09999853283271,-1.31980133087414,0.635631300872562));
#18292=CARTESIAN_POINT('Ctrl Pts',(7.09999885939544,-1.32233451509485,0.628092322434426));
#18293=CARTESIAN_POINT('Ctrl Pts',(7.09999934101855,-1.32395982399511,0.620358959365968));
#18294=CARTESIAN_POINT('Ctrl Pts',(7.09999964997549,-1.32500244522074,0.615398075635307));
#18295=CARTESIAN_POINT('Ctrl Pts',(7.09999999934316,-1.32567060646853,0.610356529630438));
#18296=CARTESIAN_POINT('Ctrl Pts',(7.09999999981141,-1.32593912630714,0.60527654995744));
#18297=CARTESIAN_POINT('',(7.09999999995537,1.22604182196549,0.7));
#18298=CARTESIAN_POINT('',(7.1,0.712777777777778,0.7));
#18299=CARTESIAN_POINT('',(7.0999999994629,1.32593912634735,0.605276549957215));
#18300=CARTESIAN_POINT('Ctrl Pts',(7.09999999981142,1.32593912630714,0.60527654995744));
#18301=CARTESIAN_POINT('Ctrl Pts',(7.09999999908198,1.32552083177145,0.613190035045322));
#18302=CARTESIAN_POINT('Ctrl Pts',(7.09999922367565,1.32413525001942,0.621012727860624));
#18303=CARTESIAN_POINT('Ctrl Pts',(7.09999888117586,1.32186630199077,0.628584136488803));
#18304=CARTESIAN_POINT('Ctrl Pts',(7.09999868987568,1.32059900146923,0.632813078704371));
#18305=CARTESIAN_POINT('Ctrl Pts',(7.09999860640034,1.3190551184949,0.636963663611311));
#18306=CARTESIAN_POINT('Ctrl Pts',(7.09999865766138,1.31724253497577,0.641005923298765));
#18307=CARTESIAN_POINT('Ctrl Pts',(7.0999987494091,1.31399834762864,0.648240816253195));
#18308=CARTESIAN_POINT('Ctrl Pts',(7.09999933613984,1.30993159792479,0.655050690394837));
#18309=CARTESIAN_POINT('Ctrl Pts',(7.09999956222935,1.30510592187917,0.661272231165006));
#18310=CARTESIAN_POINT('Ctrl Pts',(7.09999960444598,1.30420484616769,0.662433950108221));
#18311=CARTESIAN_POINT('Ctrl Pts',(7.09999963060969,1.30327718139331,0.663575086117144));
#18312=CARTESIAN_POINT('Ctrl Pts',(7.09999963056866,1.30232317316131,0.664694459428815));
#18313=CARTESIAN_POINT('Ctrl Pts',(7.09999963048683,1.30042028596585,0.666927187690779));
#18314=CARTESIAN_POINT('Ctrl Pts',(7.09999952705857,1.29841262431024,0.669073382394206));
#18315=CARTESIAN_POINT('Ctrl Pts',(7.09999938633452,1.29630755303174,0.671129253595323));
#18316=CARTESIAN_POINT('Ctrl Pts',(7.09999900634735,1.29062337821964,0.676680576924663));
#18317=CARTESIAN_POINT('Ctrl Pts',(7.09999841760642,1.2842958957007,0.681513596217188));
#18318=CARTESIAN_POINT('Ctrl Pts',(7.0999982224057,1.2774887935492,0.68557385059291));
#18319=CARTESIAN_POINT('Ctrl Pts',(7.09999809840912,1.27316474526651,0.688153029745784));
#18320=CARTESIAN_POINT('Ctrl Pts',(7.09999810738417,1.26864620899217,0.690419707112974));
#18321=CARTESIAN_POINT('Ctrl Pts',(7.09999825155258,1.26396949224645,0.69235064530212));
#18322=CARTESIAN_POINT('Ctrl Pts',(7.09999847710269,1.25665281355793,0.695371579659609));
#18323=CARTESIAN_POINT('Ctrl Pts',(7.09999903441007,1.2490339950321,0.697538299034574));
#18324=CARTESIAN_POINT('Ctrl Pts',(7.09999948258254,1.24125996729125,0.698781081437474));
#18325=CARTESIAN_POINT('Ctrl Pts',(7.09999977198436,1.23623998534067,0.699583592753232));
#18326=CARTESIAN_POINT('Ctrl Pts',(7.1,1.23115469319345,0.7));
#18327=CARTESIAN_POINT('Ctrl Pts',(7.1,1.22604182196307,0.7));
#18328=CARTESIAN_POINT('Ctrl Pts',(7.1,1.35793097395724,0.));
#18329=CARTESIAN_POINT('Ctrl Pts',(7.1,1.35259441576718,0.100972845781549));
#18330=CARTESIAN_POINT('Ctrl Pts',(7.1,1.34725763161617,0.201946637598055));
#18331=CARTESIAN_POINT('Ctrl Pts',(7.1,1.33659371676552,0.403704849408333));
#18332=CARTESIAN_POINT('Ctrl Pts',(7.0999999994629,1.33126648576411,0.504491180117376));
#18333=CARTESIAN_POINT('Ctrl Pts',(7.0999999994629,1.32593912634735,0.605276549957215));
#18334=CARTESIAN_POINT('Ctrl Pts',(7.11011156210589,-1.35766432821499,-9.27062925672982E-5));
#18335=CARTESIAN_POINT('Ctrl Pts',(7.10674110347764,-1.34708925835705,0.201697046690488));
#18336=CARTESIAN_POINT('Ctrl Pts',(7.10337058314201,-1.33651419103807,0.403486798779133));
#18337=CARTESIAN_POINT('Ctrl Pts',(7.09999999999996,-1.32593912631822,0.605276549958221));
#18338=CARTESIAN_POINT('Ctrl Pts',(5.9694837631095,-1.38835096090528,2.80675674898241E-6));
#18339=CARTESIAN_POINT('Ctrl Pts',(5.96835662351021,-1.37777563343505,0.201792740207853));
#18340=CARTESIAN_POINT('Ctrl Pts',(5.96722945517891,-1.3672003004237,0.40358267322573));
#18341=CARTESIAN_POINT('Ctrl Pts',(5.96610224583462,-1.35662497356325,0.605372606931572));
#18342=CARTESIAN_POINT('Ctrl Pts',(4.8294200007394,-1.39866452387306,3.01102374082134E-5));
#18343=CARTESIAN_POINT('Ctrl Pts',(4.83053730380309,-1.38808904115766,0.201820093264151));
#18344=CARTESIAN_POINT('Ctrl Pts',(4.83165461298617,-1.3775135517806,0.403610075973038));
#18345=CARTESIAN_POINT('Ctrl Pts',(4.83277191472125,-1.36693806692183,0.605400059795761));
#18346=CARTESIAN_POINT('Ctrl Pts',(3.68991216363982,-1.37907703205181,-6.2684699445455E-5));
#18347=CARTESIAN_POINT('Ctrl Pts',(3.69327498756969,-1.36850179198701,0.201727122618256));
#18348=CARTESIAN_POINT('Ctrl Pts',(3.69663785098144,-1.3579265529724,0.403516929334346));
#18349=CARTESIAN_POINT('Ctrl Pts',(3.70000075457889,-1.34735131503281,0.605306735438421));
#18350=CARTESIAN_POINT('Ctrl Pts',(3.69999999992215,-1.34735368792773,0.6052614572053));
#18351=CARTESIAN_POINT('Ctrl Pts',(4.83355316856959,-1.366961322855,0.605214762857233));
#18352=CARTESIAN_POINT('Ctrl Pts',(5.96724522208681,-1.35660163688233,0.605228569880684));
#18353=CARTESIAN_POINT('Ctrl Pts',(7.09999999927392,-1.32593912632169,0.605276549957417));
#18354=CARTESIAN_POINT('Ctrl Pts',(7.1,-1.22604182196307,0.7));
#18355=CARTESIAN_POINT('Ctrl Pts',(5.96696284938742,-1.25674179781664,0.7));
#18356=CARTESIAN_POINT('Ctrl Pts',(4.83327074934872,-1.26710800714677,0.7));
#18357=CARTESIAN_POINT('Ctrl Pts',(3.7,-1.24747724070879,0.7));
#18358=CARTESIAN_POINT('Ctrl Pts',(7.10078315634008,-1.25494559805327,0.7));
#18359=CARTESIAN_POINT('Ctrl Pts',(5.96739926106349,-1.28566432005869,0.700000343763215));
#18360=CARTESIAN_POINT('Ctrl Pts',(4.83328164159484,-1.29603890521481,0.700000334703603));
#18361=CARTESIAN_POINT('Ctrl Pts',(3.69949916377151,-1.27639017438114,0.7));
#18362=CARTESIAN_POINT('Ctrl Pts',(7.10214055788579,-1.30504291366416,0.676629771601708));
#18363=CARTESIAN_POINT('Ctrl Pts',(5.96815960929481,-1.33579288254824,0.676614006760374));
#18364=CARTESIAN_POINT('Ctrl Pts',(4.83329467960724,-1.3461818279488,0.676609489640654));
#18365=CARTESIAN_POINT('Ctrl Pts',(3.69863109538965,-1.3265031696486,0.676624836591801));
#18366=CARTESIAN_POINT('Ctrl Pts',(7.10267376869946,-1.32472200604796,0.626932241521275));
#18367=CARTESIAN_POINT('Ctrl Pts',(5.9684558952243,-1.35546668061705,0.626891484245174));
#18368=CARTESIAN_POINT('Ctrl Pts',(4.83330292199863,-1.36585610284781,0.626879766983475));
#18369=CARTESIAN_POINT('Ctrl Pts',(3.69829020046733,-1.34618280086838,0.626919440930842));
#18370=CARTESIAN_POINT('Ctrl Pts',(7.10270476209941,-1.32586587253612,0.605276664588022));
#18371=CARTESIAN_POINT('Ctrl Pts',(5.96847377630401,-1.35660073810322,0.605228567467576));
#18372=CARTESIAN_POINT('Ctrl Pts',(4.8333022084086,-1.36698748587873,0.605214711607465));
#18373=CARTESIAN_POINT('Ctrl Pts',(3.69827043673666,-1.34732374755196,0.60526152849799));
#18374=CARTESIAN_POINT('Ctrl Pts',(7.1,-1.22604182196307,0.7));
#18375=CARTESIAN_POINT('Ctrl Pts',(5.96696284938742,-1.25674179781664,0.7));
#18376=CARTESIAN_POINT('Ctrl Pts',(4.83327074934872,-1.26710800714677,0.7));
#18377=CARTESIAN_POINT('Ctrl Pts',(3.7,-1.24747724070879,0.7));
#18378=CARTESIAN_POINT('Origin',(5.4,-8.11656130105013E-18,0.7));
#18379=CARTESIAN_POINT('Ctrl Pts',(3.7,1.24747724070879,0.7));
#18380=CARTESIAN_POINT('Ctrl Pts',(4.83327074934871,1.26710800714677,0.7));
#18381=CARTESIAN_POINT('Ctrl Pts',(5.96696284938742,1.25674179781664,0.7));
#18382=CARTESIAN_POINT('Ctrl Pts',(7.1,1.22604182196307,0.7));
#18383=CARTESIAN_POINT('Ctrl Pts',(3.7,1.24747724070879,0.7));
#18384=CARTESIAN_POINT('Ctrl Pts',(4.83327074934871,1.26710800714677,0.7));
#18385=CARTESIAN_POINT('Ctrl Pts',(5.96696284938742,1.25674179781664,0.7));
#18386=CARTESIAN_POINT('Ctrl Pts',(7.1,1.22604182196307,0.7));
#18387=CARTESIAN_POINT('Ctrl Pts',(3.69949916377151,1.27639017438114,0.7));
#18388=CARTESIAN_POINT('Ctrl Pts',(4.83328164159484,1.29603890521481,0.700000334703603));
#18389=CARTESIAN_POINT('Ctrl Pts',(5.96739926106349,1.28566432005869,0.700000343763215));
#18390=CARTESIAN_POINT('Ctrl Pts',(7.10078315634008,1.25494559805327,0.7));
#18391=CARTESIAN_POINT('Ctrl Pts',(3.69863109538965,1.3265031696486,0.676624836591801));
#18392=CARTESIAN_POINT('Ctrl Pts',(4.83329467960724,1.3461818279488,0.676609489640654));
#18393=CARTESIAN_POINT('Ctrl Pts',(5.9681596092948,1.33579288254824,0.676614006760374));
#18394=CARTESIAN_POINT('Ctrl Pts',(7.10214055788579,1.30504291366416,0.676629771601707));
#18395=CARTESIAN_POINT('Ctrl Pts',(3.69829020046733,1.34618280086838,0.626919440930842));
#18396=CARTESIAN_POINT('Ctrl Pts',(4.83330292199863,1.36585610284781,0.626879766983475));
#18397=CARTESIAN_POINT('Ctrl Pts',(5.9684558952243,1.35546668061705,0.626891484245174));
#18398=CARTESIAN_POINT('Ctrl Pts',(7.10267376869946,1.32472200604796,0.626932241521275));
#18399=CARTESIAN_POINT('Ctrl Pts',(3.69827043673666,1.34732374755196,0.60526152849799));
#18400=CARTESIAN_POINT('Ctrl Pts',(4.83330220840859,1.36698748587873,0.605214711607465));
#18401=CARTESIAN_POINT('Ctrl Pts',(5.96847377630401,1.35660073810322,0.605228567467576));
#18402=CARTESIAN_POINT('Ctrl Pts',(7.10270476209941,1.32586587253612,0.605276664588022));
#18403=CARTESIAN_POINT('Ctrl Pts',(7.09999999927392,1.32593912632169,0.605276549957417));
#18404=CARTESIAN_POINT('Ctrl Pts',(5.96724522208681,1.35660163688233,0.605228569880684));
#18405=CARTESIAN_POINT('Ctrl Pts',(4.83355316856959,1.366961322855,0.605214762857233));
#18406=CARTESIAN_POINT('Ctrl Pts',(3.69999999992215,1.34735368792773,0.6052614572053));
#18407=CARTESIAN_POINT('Ctrl Pts',(3.68991216360307,1.37907703216746,-6.26869063400631E-5));
#18408=CARTESIAN_POINT('Ctrl Pts',(3.6932749875452,1.36850179206412,0.201727121146993));
#18409=CARTESIAN_POINT('Ctrl Pts',(3.69663785096921,1.35792655301095,0.403516928598715));
#18410=CARTESIAN_POINT('Ctrl Pts',(3.70000075457892,1.34735131503281,0.605306735438421));
#18411=CARTESIAN_POINT('Ctrl Pts',(4.8294200007272,1.39866452398872,3.01080305115927E-5));
#18412=CARTESIAN_POINT('Ctrl Pts',(4.83053730379496,1.38808904123477,0.201820091792887));
#18413=CARTESIAN_POINT('Ctrl Pts',(4.83165461298211,1.37751355181915,0.403610075237406));
#18414=CARTESIAN_POINT('Ctrl Pts',(4.83277191472127,1.36693806692183,0.605400059795761));
#18415=CARTESIAN_POINT('Ctrl Pts',(5.96948376312183,1.38835096102094,2.80454985295556E-6));
#18416=CARTESIAN_POINT('Ctrl Pts',(5.96835662351844,1.37777563351215,0.201792738736588));
#18417=CARTESIAN_POINT('Ctrl Pts',(5.96722945518303,1.36720030046225,0.403582672490098));
#18418=CARTESIAN_POINT('Ctrl Pts',(5.96610224583462,1.35662497356325,0.605372606931572));
#18419=CARTESIAN_POINT('Ctrl Pts',(7.11011156214274,1.35766432833065,-9.27084994613511E-5));
#18420=CARTESIAN_POINT('Ctrl Pts',(7.10674110350221,1.34708925843416,0.201697045219225));
#18421=CARTESIAN_POINT('Ctrl Pts',(7.10337058315429,1.33651419107662,0.403486798043502));
#18422=CARTESIAN_POINT('Ctrl Pts',(7.09999999999996,1.32593912631822,0.605276549958221));
#18423=CARTESIAN_POINT('Origin',(3.5,1.44777777777778,0.));
#18424=CARTESIAN_POINT('',(3.5,-1.34358136363184,0.605270327458634));
#18425=CARTESIAN_POINT('Ctrl Pts',(3.5,-1.34358136363184,0.605270327458634));
#18426=CARTESIAN_POINT('Ctrl Pts',(3.5,-1.34890136370362,0.504489156176152));
#18427=CARTESIAN_POINT('Ctrl Pts',(3.5,-1.35422123464986,0.403706701640381));
#18428=CARTESIAN_POINT('Ctrl Pts',(3.5,-1.3648706701715,0.201950780690867));
#18429=CARTESIAN_POINT('Ctrl Pts',(3.5,-1.3702003690246,0.100974756199658));
#18430=CARTESIAN_POINT('Ctrl Pts',(3.5,-1.37552980833516,0.));
#18431=CARTESIAN_POINT('',(3.5,-1.24369946473884,0.7));
#18432=CARTESIAN_POINT('Ctrl Pts',(3.49999999991873,-1.24369946470729,0.7));
#18433=CARTESIAN_POINT('Ctrl Pts',(3.49999999896975,-1.25160831520001,0.699999999810925));
#18434=CARTESIAN_POINT('Ctrl Pts',(3.50000040534574,-1.25945374057332,0.69900619751828));
#18435=CARTESIAN_POINT('Ctrl Pts',(3.50000075715473,-1.26709539726361,0.697119355224275));
#18436=CARTESIAN_POINT('Ctrl Pts',(3.5000009551612,-1.27139630362835,0.696057395447694));
#18437=CARTESIAN_POINT('Ctrl Pts',(3.50000113454144,-1.27563271975905,0.694711510656402));
#18438=CARTESIAN_POINT('Ctrl Pts',(3.50000124621709,-1.27977793997275,0.693092697679401));
#18439=CARTESIAN_POINT('Ctrl Pts',(3.50000144618968,-1.28720060051191,0.690193961644836));
#18440=CARTESIAN_POINT('Ctrl Pts',(3.50000138985083,-1.29425038514255,0.686454755369034));
#18441=CARTESIAN_POINT('Ctrl Pts',(3.5000011147959,-1.30078112659466,0.681956784255818));
#18442=CARTESIAN_POINT('Ctrl Pts',(3.50000096334461,-1.30437709646577,0.679480102439082));
#18443=CARTESIAN_POINT('Ctrl Pts',(3.50000075087427,-1.30781543681835,0.676772489296601));
#18444=CARTESIAN_POINT('Ctrl Pts',(3.50000056308077,-1.31106783354026,0.67384203444854));
#18445=CARTESIAN_POINT('Ctrl Pts',(3.50000037990614,-1.31424023611357,0.670983655445047));
#18446=CARTESIAN_POINT('Ctrl Pts',(3.50000021841608,-1.31721646102264,0.667930553458483));
#18447=CARTESIAN_POINT('Ctrl Pts',(3.50000022028926,-1.3199739184757,0.664694242102541));
#18448=CARTESIAN_POINT('Ctrl Pts',(3.50000022375892,-1.32508151834405,0.658699667848218));
#18449=CARTESIAN_POINT('Ctrl Pts',(3.50000072745304,-1.32944146850927,0.652077914129702));
#18450=CARTESIAN_POINT('Ctrl Pts',(3.50000090782832,-1.33299465793893,0.64499486611401));
#18451=CARTESIAN_POINT('Ctrl Pts',(3.50000092626355,-1.33335781125732,0.644270944003422));
#18452=CARTESIAN_POINT('Ctrl Pts',(3.50000094214549,-1.33371249714824,0.643542183465449));
#18453=CARTESIAN_POINT('Ctrl Pts',(3.5000009551778,-1.33405862411533,0.642808750463418));
#18454=CARTESIAN_POINT('Ctrl Pts',(3.50000108270827,-1.3374457225345,0.635631587173848));
#18455=CARTESIAN_POINT('Ctrl Pts',(3.5000008470667,-1.33997810357527,0.628091493562486));
#18456=CARTESIAN_POINT('Ctrl Pts',(3.50000049017339,-1.34160279315579,0.620357239364781));
#18457=CARTESIAN_POINT('Ctrl Pts',(3.50000026118253,-1.3426452308862,0.615394766232079));
#18458=CARTESIAN_POINT('Ctrl Pts',(3.5,-1.34331313055125,0.610351689051435));
#18459=CARTESIAN_POINT('Ctrl Pts',(3.5,-1.34358136363184,0.605270327458634));
#18460=CARTESIAN_POINT('',(3.5,0.723888888888889,0.7));
#18461=CARTESIAN_POINT('Ctrl Pts',(3.5,1.37552980833516,0.));
#18462=CARTESIAN_POINT('Ctrl Pts',(3.5,1.37020035376703,0.10097504527886));
#18463=CARTESIAN_POINT('Ctrl Pts',(3.5,1.36487063968137,0.201951358354439));
#18464=CARTESIAN_POINT('Ctrl Pts',(3.5,1.35422120417274,0.403707279015233));
#18465=CARTESIAN_POINT('Ctrl Pts',(3.5,1.34890134846466,0.504489444860456));
#18466=CARTESIAN_POINT('Ctrl Pts',(3.5,1.34358136363184,0.605270327458635));
#18467=CARTESIAN_POINT('Ctrl Pts',(3.50000000097418,-1.37552980835478,3.46944695195361E-18));
#18468=CARTESIAN_POINT('Ctrl Pts',(3.50374047168104,-1.36494504174376,0.201972406882836));
#18469=CARTESIAN_POINT('Ctrl Pts',(3.50748098869546,-1.35436027657305,0.403944812985359));
#18470=CARTESIAN_POINT('Ctrl Pts',(3.51122155284351,-1.34377551287676,0.605917218294091));
#18471=CARTESIAN_POINT('Ctrl Pts',(2.69119625874569,-1.35924722858667,-7.54309614812119E-5));
#18472=CARTESIAN_POINT('Ctrl Pts',(2.69653217397324,-1.34866266892899,0.20189683354744));
#18473=CARTESIAN_POINT('Ctrl Pts',(2.70186816749714,-1.3380781117335,0.403869096002786));
#18474=CARTESIAN_POINT('Ctrl Pts',(2.7072042346663,-1.32749355863083,0.605841357314298));
#18475=CARTESIAN_POINT('Ctrl Pts',(1.88267190563219,-1.32763345268679,-0.000212792412547521));
#18476=CARTESIAN_POINT('Ctrl Pts',(1.88960380459144,-1.31704931403188,0.201759213581099));
#18477=CARTESIAN_POINT('Ctrl Pts',(1.89653581411498,-1.30646518166523,0.403731216009517));
#18478=CARTESIAN_POINT('Ctrl Pts',(1.90346792975642,-1.29588105699583,0.605703215867581));
#18479=CARTESIAN_POINT('Ctrl Pts',(1.07441451989529,-1.27728918272486,-0.000429194541766893));
#18480=CARTESIAN_POINT('Ctrl Pts',(1.08294287068452,-1.26670581246828,0.201542410257184));
#18481=CARTESIAN_POINT('Ctrl Pts',(1.09147136321593,-1.25612245578053,0.403514009799157));
#18482=CARTESIAN_POINT('Ctrl Pts',(1.09999999999989,-1.24553911298205,0.605485603995245));
#18483=CARTESIAN_POINT('Ctrl Pts',(1.09999999916631,-1.24553911263844,0.605485603997431));
#18484=CARTESIAN_POINT('Ctrl Pts',(1.89930203168262,-1.29563783986497,0.605377360150118));
#18485=CARTESIAN_POINT('Ctrl Pts',(2.69958486793449,-1.32722445934619,0.605308375488923));
#18486=CARTESIAN_POINT('Ctrl Pts',(3.5,-1.34358136363184,0.605270327458634));
#18487=CARTESIAN_POINT('Ctrl Pts',(3.50204003610941,-1.24374118183538,0.7));
#18488=CARTESIAN_POINT('Ctrl Pts',(2.70080437300401,-1.2273695200909,0.7));
#18489=CARTESIAN_POINT('Ctrl Pts',(1.89984199608574,-1.1957170361627,0.7));
#18490=CARTESIAN_POINT('Ctrl Pts',(1.1,-1.14549341399196,0.7));
#18491=CARTESIAN_POINT('Ctrl Pts',(3.50144932661635,-1.27265074030048,0.7));
#18492=CARTESIAN_POINT('Ctrl Pts',(2.6998452019678,-1.25626413437997,0.699999727319846));
#18493=CARTESIAN_POINT('Ctrl Pts',(1.89847848223078,-1.22458382597074,0.70000077422621));
#18494=CARTESIAN_POINT('Ctrl Pts',(1.09819048660397,-1.17431102498992,0.7));
#18495=CARTESIAN_POINT('Ctrl Pts',(3.50042536655637,-1.322763754511,0.676632802377821));
#18496=CARTESIAN_POINT('Ctrl Pts',(2.69818680938114,-1.3063522351595,0.67664530655333));
#18497=CARTESIAN_POINT('Ctrl Pts',(1.89610976425884,-1.27462253270773,0.67666760713801));
#18498=CARTESIAN_POINT('Ctrl Pts',(1.09505363188407,-1.22426736091617,0.676703190608825));
#18499=CARTESIAN_POINT('Ctrl Pts',(3.50002334924346,-1.34243864233338,0.626926882269943));
#18500=CARTESIAN_POINT('Ctrl Pts',(2.6975332861013,-1.32603127467068,0.626959208652505));
#18501=CARTESIAN_POINT('Ctrl Pts',(1.89518106151152,-1.29430885982199,0.62701751976321));
#18502=CARTESIAN_POINT('Ctrl Pts',(1.09381704710221,-1.24396073223232,0.627109609335854));
#18503=CARTESIAN_POINT('Ctrl Pts',(3.5,-1.34358136363184,0.605270327458634));
#18504=CARTESIAN_POINT('Ctrl Pts',(2.69749615303,-1.32718177535833,0.605308474776761));
#18505=CARTESIAN_POINT('Ctrl Pts',(1.89512529323683,-1.29547288309274,0.605377720397184));
#18506=CARTESIAN_POINT('Ctrl Pts',(1.09374258853658,-1.24514653057163,0.605486452199395));
#18507=CARTESIAN_POINT('Ctrl Pts',(3.49999999991875,-1.24369946470729,0.7));
#18508=CARTESIAN_POINT('Ctrl Pts',(3.26917843083003,-1.23897560807887,0.7));
#18509=CARTESIAN_POINT('Ctrl Pts',(3.03837960179139,-1.23298334389983,0.7));
#18510=CARTESIAN_POINT('Ctrl Pts',(2.80762376541487,-1.22564400623233,0.7));
#18511=CARTESIAN_POINT('Ctrl Pts',(2.57739190516312,-1.2178709162388,0.7));
#18512=CARTESIAN_POINT('Ctrl Pts',(2.08463535466707,-1.20026407570248,0.7));
#18513=CARTESIAN_POINT('Ctrl Pts',(1.59210562457525,-1.17639367564078,0.7));
#18514=CARTESIAN_POINT('Ctrl Pts',(1.1,-1.14549341399196,0.7));
#18515=CARTESIAN_POINT('Origin',(5.4,-8.11656130105013E-18,0.7));
#18516=CARTESIAN_POINT('Ctrl Pts',(1.0744145198953,1.27728918272486,-0.000429194541767127));
#18517=CARTESIAN_POINT('Ctrl Pts',(1.08294287068452,1.26670581246828,0.201542410257184));
#18518=CARTESIAN_POINT('Ctrl Pts',(1.09147136321593,1.25612245578053,0.403514009799157));
#18519=CARTESIAN_POINT('Ctrl Pts',(1.0999999999999,1.24553911298205,0.605485603995245));
#18520=CARTESIAN_POINT('Ctrl Pts',(1.88267190563235,1.3276334526868,-0.000212792412547728));
#18521=CARTESIAN_POINT('Ctrl Pts',(1.8896038045916,1.31704931403189,0.201759213581098));
#18522=CARTESIAN_POINT('Ctrl Pts',(1.89653581411514,1.30646518166524,0.403731216009517));
#18523=CARTESIAN_POINT('Ctrl Pts',(1.90346792975658,1.29588105699584,0.605703215867581));
#18524=CARTESIAN_POINT('Ctrl Pts',(2.69119625874601,1.35924722858668,-7.54309614812134E-5));
#18525=CARTESIAN_POINT('Ctrl Pts',(2.69653217397356,1.348662668929,0.201896833547441));
#18526=CARTESIAN_POINT('Ctrl Pts',(2.70186816749745,1.33807811173351,0.403869096002786));
#18527=CARTESIAN_POINT('Ctrl Pts',(2.70720423466661,1.32749355863085,0.605841357314298));
#18528=CARTESIAN_POINT('Ctrl Pts',(3.50000000097466,1.37552980835479,-3.81639164714898E-17));
#18529=CARTESIAN_POINT('Ctrl Pts',(3.50374047168151,1.36494504174377,0.201972406882836));
#18530=CARTESIAN_POINT('Ctrl Pts',(3.50748098869594,1.35436027657306,0.403944812985359));
#18531=CARTESIAN_POINT('Ctrl Pts',(3.51122155284398,1.34377551287677,0.605917218294091));
#18532=CARTESIAN_POINT('Origin',(0.9,1.34328341716202,0.));
#18533=CARTESIAN_POINT('',(0.9,-1.23261418131727,0.605513513251856));
#18534=CARTESIAN_POINT('Ctrl Pts',(0.9,-1.23261418131727,0.605513513251856));
#18535=CARTESIAN_POINT('Ctrl Pts',(0.9,-1.23820195798151,0.504544236118289));
#18536=CARTESIAN_POINT('Ctrl Pts',(0.9,-1.24378834611607,0.403573587101897));
#18537=CARTESIAN_POINT('Ctrl Pts',(0.9,-1.25495246062481,0.201736610752668));
#18538=CARTESIAN_POINT('Ctrl Pts',(0.9,-1.26053033259331,0.100867703930409));
#18539=CARTESIAN_POINT('Ctrl Pts',(0.9,-1.266106713614,0.));
#18540=CARTESIAN_POINT('',(0.9,-1.13254484134404,0.7));
#18541=CARTESIAN_POINT('Ctrl Pts',(0.899999999937205,-1.13254484130906,
0.7));
#18542=CARTESIAN_POINT('Ctrl Pts',(0.899999996287105,-1.14047016437301,
0.699999998205918));
#18543=CARTESIAN_POINT('Ctrl Pts',(0.900001280561548,-1.14833327216777,
0.699006663725481));
#18544=CARTESIAN_POINT('Ctrl Pts',(0.900002371513522,-1.15599299513142,
0.697119896446058));
#18545=CARTESIAN_POINT('Ctrl Pts',(0.900002982478546,-1.16028266409831,
0.696063251566776));
#18546=CARTESIAN_POINT('Ctrl Pts',(0.900003528700818,-1.16450859688491,
0.694725368779139));
#18547=CARTESIAN_POINT('Ctrl Pts',(0.900003857331964,-1.16864431737637,
0.693116947675672));
#18548=CARTESIAN_POINT('Ctrl Pts',(0.900004447924614,-1.17607674172948,
0.690226407030055));
#18549=CARTESIAN_POINT('Ctrl Pts',(0.900004211500339,-1.18313828052408,
0.686496282267003));
#18550=CARTESIAN_POINT('Ctrl Pts',(0.900003280035406,-1.18968205680082,
0.682006679400108));
#18551=CARTESIAN_POINT('Ctrl Pts',(0.900002768383153,-1.19327654302499,
0.679540547464272));
#18552=CARTESIAN_POINT('Ctrl Pts',(0.900002064672634,-1.19671453445753,
0.676844382327844));
#18553=CARTESIAN_POINT('Ctrl Pts',(0.900001450170085,-1.19996775918788,
0.673925988054463));
#18554=CARTESIAN_POINT('Ctrl Pts',(0.900000850201302,-1.20314404102283,
0.67107661751105));
#18555=CARTESIAN_POINT('Ctrl Pts',(0.900000329673364,-1.20612495630093,
0.668032594545539));
#18556=CARTESIAN_POINT('Ctrl Pts',(0.900000346081477,-1.20888784276431,
0.664805176146368));
#18557=CARTESIAN_POINT('Ctrl Pts',(0.900000376514472,-1.21401231436848,
0.658819112599938));
#18558=CARTESIAN_POINT('Ctrl Pts',(0.900002057232535,-1.21838968018573,
0.652203523053766));
#18559=CARTESIAN_POINT('Ctrl Pts',(0.900002698394847,-1.22195969054856,
0.645123732731769));
#18560=CARTESIAN_POINT('Ctrl Pts',(0.900002763240662,-1.22232075393107,
0.644407697543824));
#18561=CARTESIAN_POINT('Ctrl Pts',(0.90000282009371,-1.22267351953901,0.643686895083047));
#18562=CARTESIAN_POINT('Ctrl Pts',(0.900002868017411,-1.22301789747605,
0.642961485862499));
#18563=CARTESIAN_POINT('Ctrl Pts',(0.900003341628975,-1.22642125256928,
0.635792544708285));
#18564=CARTESIAN_POINT('Ctrl Pts',(0.900002645022176,-1.22896979279554,
0.628258742918086));
#18565=CARTESIAN_POINT('Ctrl Pts',(0.900001532827652,-1.23061007098772,
0.6205286650049));
#18566=CARTESIAN_POINT('Ctrl Pts',(0.900000822323555,-1.23165793118585,
0.61559045329652));
#18567=CARTESIAN_POINT('Ctrl Pts',(0.900000000000001,-1.23233426661673,
0.610571479357261));
#18568=CARTESIAN_POINT('Ctrl Pts',(0.900000000000001,-1.23261418131727,
0.605513513251856));
#18569=CARTESIAN_POINT('',(0.9,1.13254484134404,0.7));
#18570=CARTESIAN_POINT('',(0.9,0.671641708581009,0.7));
#18571=CARTESIAN_POINT('',(0.9,1.23261418131727,0.605513513251856));
#18572=CARTESIAN_POINT('Ctrl Pts',(0.9,1.23261418131727,0.605513513251856));
#18573=CARTESIAN_POINT('Ctrl Pts',(0.9,1.23217633603244,0.613425232807268));
#18574=CARTESIAN_POINT('Ctrl Pts',(0.900001832787994,1.23077105609892,0.621244170085157));
#18575=CARTESIAN_POINT('Ctrl Pts',(0.900002580745575,1.22848219166492,0.628809599741497));
#18576=CARTESIAN_POINT('Ctrl Pts',(0.900002993068559,1.22722042035689,0.632980157827643));
#18577=CARTESIAN_POINT('Ctrl Pts',(0.90000314174678,1.22568915198244,0.637073706995481));
#18578=CARTESIAN_POINT('Ctrl Pts',(0.900002971484041,1.2238959908032,0.641061424759933));
#18579=CARTESIAN_POINT('Ctrl Pts',(0.900002662567364,1.22064256379503,0.648296551655426));
#18580=CARTESIAN_POINT('Ctrl Pts',(0.900001146653719,1.21656554418039,0.655104870690721));
#18581=CARTESIAN_POINT('Ctrl Pts',(0.900000540233788,1.21172928299109,0.66132323772617));
#18582=CARTESIAN_POINT('Ctrl Pts',(0.900000424918953,1.21080963534652,0.66250570210793));
#18583=CARTESIAN_POINT('Ctrl Pts',(0.900000351402035,1.20986240082127,0.663666762843393));
#18584=CARTESIAN_POINT('Ctrl Pts',(0.900000346234225,1.20888784277449,0.664805176146358));
#18585=CARTESIAN_POINT('Ctrl Pts',(0.900000336405833,1.20703438079614,0.666970266034709));
#18586=CARTESIAN_POINT('Ctrl Pts',(0.900000571869483,1.20508211779724,0.669053482241208));
#18587=CARTESIAN_POINT('Ctrl Pts',(0.900000903580486,1.20303784749416,0.671051418948595));
#18588=CARTESIAN_POINT('Ctrl Pts',(0.900001825932764,1.19735357006848,0.676606861644505));
#18589=CARTESIAN_POINT('Ctrl Pts',(0.900003332967427,1.19102482074992,0.681443262092019));
#18590=CARTESIAN_POINT('Ctrl Pts',(0.900003895332687,1.18421635668109,0.685507797106414));
#18591=CARTESIAN_POINT('Ctrl Pts',(0.900004254598985,1.17986677848026,0.688104419886002));
#18592=CARTESIAN_POINT('Ctrl Pts',(0.9000042929279,1.17532044218795,0.69038534615497));
#18593=CARTESIAN_POINT('Ctrl Pts',(0.900003997675654,1.17061445353731,0.692327416690341));
#18594=CARTESIAN_POINT('Ctrl Pts',(0.900003537640084,1.16328200409216,0.695353376818313));
#18595=CARTESIAN_POINT('Ctrl Pts',(0.900002259964378,1.15564663185935,0.697524398440697));
#18596=CARTESIAN_POINT('Ctrl Pts',(0.900001215101098,1.14785635641255,0.698771715080855));
#18597=CARTESIAN_POINT('Ctrl Pts',(0.900000537649455,1.14280542295857,0.699580430175527));
#18598=CARTESIAN_POINT('Ctrl Pts',(0.899999997568109,1.13768876957788,0.699999998835552));
#18599=CARTESIAN_POINT('Ctrl Pts',(0.899999999937205,1.13254484130906,0.7));
#18600=CARTESIAN_POINT('Ctrl Pts',(0.9,1.266106713614,0.));
#18601=CARTESIAN_POINT('Ctrl Pts',(0.9,1.26053025554556,0.100869097599589));
#18602=CARTESIAN_POINT('Ctrl Pts',(0.9,1.25495230648558,0.201739398169819));
#18603=CARTESIAN_POINT('Ctrl Pts',(0.9,1.24378819189631,0.403576374532447));
#18604=CARTESIAN_POINT('Ctrl Pts',(0.9,1.23820188085298,0.504545629805417));
#18605=CARTESIAN_POINT('Ctrl Pts',(0.9,1.23261418131727,0.605513513251856));
#18606=CARTESIAN_POINT('Ctrl Pts',(0.900000000000002,-1.266106713614,-8.15320033709099E-17));
#18607=CARTESIAN_POINT('Ctrl Pts',(0.908871090277923,-1.25552568177643,
0.201930159665972));
#18608=CARTESIAN_POINT('Ctrl Pts',(0.917742329685194,-1.24494466498547,
0.403860313587921));
#18609=CARTESIAN_POINT('Ctrl Pts',(0.926613720860141,-1.23436366359623,
0.605790461668883));
#18610=CARTESIAN_POINT('Ctrl Pts',(0.697441255022372,-1.25280938151844,
-5.71013218131409E-5));
#18611=CARTESIAN_POINT('Ctrl Pts',(0.706712389899261,-1.24222855501813,
0.201872952723963));
#18612=CARTESIAN_POINT('Ctrl Pts',(0.71598368260269,-1.23164774534186,0.403803000441224));
#18613=CARTESIAN_POINT('Ctrl Pts',(0.725255135891715,-1.22106695288555,
0.605733041729342));
#18614=CARTESIAN_POINT('Ctrl Pts',(0.494899146035781,-1.23832021354117,
-0.000119230777047918));
#18615=CARTESIAN_POINT('Ctrl Pts',(0.504570354086872,-1.2277396148863,0.201810708652083));
#18616=CARTESIAN_POINT('Ctrl Pts',(0.514241728780064,-1.21715903502506,
0.403740641123913));
#18617=CARTESIAN_POINT('Ctrl Pts',(0.523913273026478,-1.20657847439907,
0.605670566527588));
#18618=CARTESIAN_POINT('Ctrl Pts',(0.292373353339556,-1.22258574808743,
-0.000186633859775947));
#18619=CARTESIAN_POINT('Ctrl Pts',(0.302444661323169,-1.21200540195431,
0.201743181663441));
#18620=CARTESIAN_POINT('Ctrl Pts',(0.312516144861689,-1.20142507679253,
0.403672989556125));
#18621=CARTESIAN_POINT('Ctrl Pts',(0.322587807049886,-1.190844773096,0.605602789690272));
#18622=CARTESIAN_POINT('',(0.32407846024449,-1.19096124572524,0.605603291426262));
#18623=CARTESIAN_POINT('Ctrl Pts',(0.292382661757373,-1.22257596919059,
-1.26634813746307E-16));
#18624=CARTESIAN_POINT('Ctrl Pts',(0.302948004341657,-1.21203750712027,
0.201867748891544));
#18625=CARTESIAN_POINT('Ctrl Pts',(0.313513270922098,-1.20149926476964,
0.403735512620674));
#18626=CARTESIAN_POINT('Ctrl Pts',(0.324078460244491,-1.19096124572524,
0.605603291426262));
#18627=CARTESIAN_POINT('Ctrl Pts',(0.324078460244487,-1.19096124572524,
0.605603291426262));
#18628=CARTESIAN_POINT('Ctrl Pts',(0.515976798438381,-1.20595780001216,
0.605571001180369));
#18629=CARTESIAN_POINT('Ctrl Pts',(0.707956283694857,-1.21982772882273,
0.605541108414459));
#18630=CARTESIAN_POINT('Ctrl Pts',(0.900000000000001,-1.23261418131727,
0.605513513251856));
#18631=CARTESIAN_POINT('Ctrl Pts',(0.906632491847682,-1.13298681949577,
0.7));
#18632=CARTESIAN_POINT('Ctrl Pts',(0.714963137593258,-1.12022681655782,
0.7));
#18633=CARTESIAN_POINT('Ctrl Pts',(0.52336552158394,-1.10638609587519,0.7));
#18634=CARTESIAN_POINT('Ctrl Pts',(0.331856371369197,-1.09142177001972,
0.7));
#18635=CARTESIAN_POINT('Ctrl Pts',(0.904714827274509,-1.16179226195561,
0.7));
#18636=CARTESIAN_POINT('Ctrl Pts',(0.712937153454425,-1.14901967286075,
0.69999980360337));
#18637=CARTESIAN_POINT('Ctrl Pts',(0.521230340369869,-1.13516557394852,
0.700000229443053));
#18638=CARTESIAN_POINT('Ctrl Pts',(0.329608751265076,-1.12018616744754,
0.7));
#18639=CARTESIAN_POINT('Ctrl Pts',(0.901389714107723,-1.21173913866089,
0.676722045797292));
#18640=CARTESIAN_POINT('Ctrl Pts',(0.709425477581998,-1.19894546296063,
0.676731074746188));
#18641=CARTESIAN_POINT('Ctrl Pts',(0.517526696841433,-1.18506766126723,
0.67674067107047));
#18642=CARTESIAN_POINT('Ctrl Pts',(0.325711429829026,-1.17006296935233,
0.676751229163451));
#18643=CARTESIAN_POINT('Ctrl Pts',(0.900079298017777,-1.23142303740181,
0.627132481749528));
#18644=CARTESIAN_POINT('Ctrl Pts',(0.708040181852795,-1.21863106773591,
0.627155851652593));
#18645=CARTESIAN_POINT('Ctrl Pts',(0.516066269599777,-1.20475540724405,
0.627181012790208));
#18646=CARTESIAN_POINT('Ctrl Pts',(0.324172915772929,-1.18975243096407,
0.627208352638976));
#18647=CARTESIAN_POINT('Ctrl Pts',(0.900000000000001,-1.23261418131727,
0.605513513251856));
#18648=CARTESIAN_POINT('Ctrl Pts',(0.707956283694857,-1.21982772882273,
0.605541108414459));
#18649=CARTESIAN_POINT('Ctrl Pts',(0.515976798438381,-1.20595780001216,
0.605571001180369));
#18650=CARTESIAN_POINT('Ctrl Pts',(0.324078460244487,-1.19096124572524,
0.605603291426262));
#18651=CARTESIAN_POINT('',(0.3318563713692,-1.09142177001972,0.7));
#18652=CARTESIAN_POINT('Origin',(0.3318563713692,-1.09142177001972,0.6));
#18653=CARTESIAN_POINT('Ctrl Pts',(0.899999999937167,-1.13254484130906,
0.7));
#18654=CARTESIAN_POINT('Ctrl Pts',(0.710543123935439,-1.11990737114256,
0.7));
#18655=CARTESIAN_POINT('Ctrl Pts',(0.521156529292483,-1.10621348751457,
0.7));
#18656=CARTESIAN_POINT('Ctrl Pts',(0.331856371369197,-1.09142177001972,
0.7));
#18657=CARTESIAN_POINT('Origin',(5.4,-8.11656130105013E-18,0.7));
#18658=CARTESIAN_POINT('',(0.3318563713692,1.09142177001972,0.7));
#18659=CARTESIAN_POINT('',(0.3318563713692,-0.7,0.7));
#18660=CARTESIAN_POINT('Ctrl Pts',(0.3318563713692,1.09142177001972,0.7));
#18661=CARTESIAN_POINT('Ctrl Pts',(0.521156529292483,1.10621348751457,0.7));
#18662=CARTESIAN_POINT('Ctrl Pts',(0.710543123935438,1.11990737114256,0.7));
#18663=CARTESIAN_POINT('Ctrl Pts',(0.899999999937165,1.13254484130906,0.7));
#18664=CARTESIAN_POINT('Ctrl Pts',(0.292373353339556,1.22258574808743,-0.000186633859776018));
#18665=CARTESIAN_POINT('Ctrl Pts',(0.30244466132317,1.21200540195431,0.20174318166344));
#18666=CARTESIAN_POINT('Ctrl Pts',(0.31251614486169,1.20142507679253,0.403672989556124));
#18667=CARTESIAN_POINT('Ctrl Pts',(0.322587807049886,1.190844773096,0.605602789690271));
#18668=CARTESIAN_POINT('Ctrl Pts',(0.494899146035781,1.23832021354117,-0.000119230777047989));
#18669=CARTESIAN_POINT('Ctrl Pts',(0.504570354086872,1.2277396148863,0.201810708652083));
#18670=CARTESIAN_POINT('Ctrl Pts',(0.514241728780064,1.21715903502506,0.403740641123914));
#18671=CARTESIAN_POINT('Ctrl Pts',(0.523913273026478,1.20657847439907,0.605670566527587));
#18672=CARTESIAN_POINT('Ctrl Pts',(0.697441255022371,1.25280938151844,-5.71013218130602E-5));
#18673=CARTESIAN_POINT('Ctrl Pts',(0.70671238989926,1.24222855501813,0.201872952723963));
#18674=CARTESIAN_POINT('Ctrl Pts',(0.715983682602689,1.23164774534186,0.403803000441224));
#18675=CARTESIAN_POINT('Ctrl Pts',(0.725255135891714,1.22106695288555,0.605733041729342));
#18676=CARTESIAN_POINT('Ctrl Pts',(0.9,1.266106713614,1.73472347597681E-18));
#18677=CARTESIAN_POINT('Ctrl Pts',(0.908871090277921,1.25552568177643,0.201930159665973));
#18678=CARTESIAN_POINT('Ctrl Pts',(0.917742329685192,1.24494466498547,0.403860313587921));
#18679=CARTESIAN_POINT('Ctrl Pts',(0.92661372086014,1.23436366359623,0.605790461668883));
#18680=CARTESIAN_POINT('',(0.32407846024449,1.19096124572524,0.605603291426262));
#18681=CARTESIAN_POINT('Ctrl Pts',(0.9,1.23261418131727,0.605513513251856));
#18682=CARTESIAN_POINT('Ctrl Pts',(0.707956283694857,1.21982772882273,0.605541108414459));
#18683=CARTESIAN_POINT('Ctrl Pts',(0.515976798438382,1.20595780001216,0.60557100118037));
#18684=CARTESIAN_POINT('Ctrl Pts',(0.32407846024449,1.19096124572524,0.605603291426262));
#18685=CARTESIAN_POINT('Ctrl Pts',(0.324078460244491,1.19096124572524,0.605603291426262));
#18686=CARTESIAN_POINT('Ctrl Pts',(0.313513270922098,1.20149926476964,0.403735512620674));
#18687=CARTESIAN_POINT('Ctrl Pts',(0.302948004341658,1.21203750712026,0.201867748891544));
#18688=CARTESIAN_POINT('Ctrl Pts',(0.292382661757373,1.22257596919059,3.4477629085039E-17));
#18689=CARTESIAN_POINT('Ctrl Pts',(0.3318563713692,1.09142177001972,0.7));
#18690=CARTESIAN_POINT('Ctrl Pts',(0.523365521583941,1.10638609587519,0.7));
#18691=CARTESIAN_POINT('Ctrl Pts',(0.714963137593258,1.12022681655782,0.7));
#18692=CARTESIAN_POINT('Ctrl Pts',(0.906632491847681,1.13298681949577,0.7));
#18693=CARTESIAN_POINT('Ctrl Pts',(0.329608751265078,1.12018616744754,0.7));
#18694=CARTESIAN_POINT('Ctrl Pts',(0.52123034036987,1.13516557394852,0.700000229443053));
#18695=CARTESIAN_POINT('Ctrl Pts',(0.712937153454426,1.14901967286075,0.699999803603371));
#18696=CARTESIAN_POINT('Ctrl Pts',(0.904714827274509,1.16179226195561,0.700000000000001));
#18697=CARTESIAN_POINT('Ctrl Pts',(0.325711429829028,1.17006296935233,0.676751229163452));
#18698=CARTESIAN_POINT('Ctrl Pts',(0.517526696841433,1.18506766126723,0.67674067107047));
#18699=CARTESIAN_POINT('Ctrl Pts',(0.709425477581997,1.19894546296063,0.676731074746189));
#18700=CARTESIAN_POINT('Ctrl Pts',(0.901389714107722,1.21173913866089,0.676722045797292));
#18701=CARTESIAN_POINT('Ctrl Pts',(0.324172915772932,1.18975243096407,0.627208352638976));
#18702=CARTESIAN_POINT('Ctrl Pts',(0.516066269599778,1.20475540724405,0.627181012790208));
#18703=CARTESIAN_POINT('Ctrl Pts',(0.708040181852794,1.21863106773591,0.627155851652593));
#18704=CARTESIAN_POINT('Ctrl Pts',(0.900079298017776,1.23142303740181,0.627132481749528));
#18705=CARTESIAN_POINT('Ctrl Pts',(0.32407846024449,1.19096124572524,0.605603291426262));
#18706=CARTESIAN_POINT('Ctrl Pts',(0.515976798438382,1.20595780001216,0.60557100118037));
#18707=CARTESIAN_POINT('Ctrl Pts',(0.707956283694857,1.21982772882273,0.605541108414459));
#18708=CARTESIAN_POINT('Ctrl Pts',(0.9,1.23261418131727,0.605513513251856));
#18709=CARTESIAN_POINT('Origin',(0.331856371369202,1.09142177001972,0.6));
#18710=CARTESIAN_POINT('Origin',(0.331856371369202,1.09142177001972,0.6));
#18711=CARTESIAN_POINT('Origin',(0.331856371369201,1.09142177001972,0.6));
#18712=CARTESIAN_POINT('Origin',(0.331856371369202,1.09142177001972,0.6));
#18713=CARTESIAN_POINT('Origin',(10.4681436286308,1.08420482079361,0.6));
#18714=CARTESIAN_POINT('Origin',(10.4681436276939,1.08420482084454,0.6));
#18715=CARTESIAN_POINT('',(10.5680065821063,1.08420482079361,0.605233595624295));
#18716=CARTESIAN_POINT('Origin',(10.4681436286308,1.08420482079361,0.6));
#18717=CARTESIAN_POINT('Origin',(10.4681436286308,1.08420482079361,0.6));
#18718=CARTESIAN_POINT('Origin',(0.3318563713692,-1.09142177001972,0.6));
#18719=CARTESIAN_POINT('Origin',(0.331856371369201,-1.09142177001972,0.6));
#18720=CARTESIAN_POINT('Origin',(0.3318563713692,-1.09142177001972,0.6));
#18721=CARTESIAN_POINT('Origin',(0.3318563713692,-0.7,0.6));
#18722=CARTESIAN_POINT('Ctrl Pts',(0.2922895713475,-1.22266882276207,-0.00177864096060679));
#18723=CARTESIAN_POINT('Ctrl Pts',(0.302885944515497,-1.21209940820877,
0.200681988163859));
#18724=CARTESIAN_POINT('Ctrl Pts',(0.313482241236256,-1.20153021465708,
0.403142632212487));
#18725=CARTESIAN_POINT('Ctrl Pts',(0.324078460244491,-1.19096124572524,
0.605603291426262));
#18726=CARTESIAN_POINT('Ctrl Pts',(0.264022491930188,-1.22039553779506,
-0.000415890128406236));
#18727=CARTESIAN_POINT('Ctrl Pts',(0.274621881512248,-1.20982222712748,
0.202044379074236));
#18728=CARTESIAN_POINT('Ctrl Pts',(0.285221154833576,-1.19924944554801,
0.404504681968985));
#18729=CARTESIAN_POINT('Ctrl Pts',(0.29582042516239,-1.18867654001483,0.606964977361795));
#18730=CARTESIAN_POINT('Ctrl Pts',(0.216712469170969,-1.1940874043406,0.000690255297866666));
#18731=CARTESIAN_POINT('Ctrl Pts',(0.227319688237882,-1.18351239299796,
0.203150045648192));
#18732=CARTESIAN_POINT('Ctrl Pts',(0.237926932441998,-1.17293746916702,
0.405609838636422));
#18733=CARTESIAN_POINT('Ctrl Pts',(0.248534117816369,-1.1623628476683,0.608069650238703));
#18734=CARTESIAN_POINT('Ctrl Pts',(0.200219987929043,-1.14439035743082,
-0.00103956457010847));
#18735=CARTESIAN_POINT('Ctrl Pts',(0.210830491339948,-1.13382006821851,
0.201420337884579));
#18736=CARTESIAN_POINT('Ctrl Pts',(0.221440906577676,-1.12324995278282,
0.403880253819325));
#18737=CARTESIAN_POINT('Ctrl Pts',(0.232051411471599,-1.11268010558856,
0.606340179010355));
#18738=CARTESIAN_POINT('Ctrl Pts',(0.200161975173303,-1.12312592850316,
-0.00214651389202307));
#18739=CARTESIAN_POINT('Ctrl Pts',(0.210772455448684,-1.11255764422181,
0.200313510564959));
#18740=CARTESIAN_POINT('Ctrl Pts',(0.221382936352032,-1.1019895901204,0.402773547004277));
#18741=CARTESIAN_POINT('Ctrl Pts',(0.231993417893744,-1.09142177001972,
0.605233595624295));
#18742=CARTESIAN_POINT('Origin',(10.4681436286308,-1.08420482109828,0.6));
#18743=CARTESIAN_POINT('',(10.5680065821063,-1.08420482079361,0.605233595624295));
#18744=CARTESIAN_POINT('Origin',(10.4681436286308,-1.08420482099672,0.600000000000001));
#18745=CARTESIAN_POINT('Origin',(10.4681436286308,-1.08420482109828,0.6));
#18746=CARTESIAN_POINT('Origin',(10.4681436286308,0.7,0.6));
#18747=CARTESIAN_POINT('',(10.5680065821063,0.7,0.605233595624295));
#18748=CARTESIAN_POINT('Ctrl Pts',(10.599839982685,-1.11594741464673,-0.00218387205330164));
#18749=CARTESIAN_POINT('Ctrl Pts',(10.5892288496247,-1.10536637943871,0.200288608282177));
#18750=CARTESIAN_POINT('Ctrl Pts',(10.5786177161011,-1.0947855138519,0.402761097457634));
#18751=CARTESIAN_POINT('Ctrl Pts',(10.5680065821063,-1.08420482079362,0.605233595624295));
#18752=CARTESIAN_POINT('Ctrl Pts',(10.5997613205547,-1.14474784499259,-0.000682909193257743));
#18753=CARTESIAN_POINT('Ctrl Pts',(10.5891501209488,-1.13416481604349,0.201789447273867));
#18754=CARTESIAN_POINT('Ctrl Pts',(10.5785391399155,-1.12358205581644,0.404261829287571));
#18755=CARTESIAN_POINT('Ctrl Pts',(10.5679279386544,-1.11299934606825,0.606734202078189));
#18756=CARTESIAN_POINT('Ctrl Pts',(10.5764119435127,-1.19466846760808,0.000702210001053139));
#18757=CARTESIAN_POINT('Ctrl Pts',(10.5658041809617,-1.18408222297768,0.203174550667819));
#18758=CARTESIAN_POINT('Ctrl Pts',(10.5551963844732,-1.17349608774572,0.405646894856767));
#18759=CARTESIAN_POINT('Ctrl Pts',(10.544588659013,-1.16291012508165,0.608119251464957));
#18760=CARTESIAN_POINT('Ctrl Pts',(10.5269342003857,-1.21442651155969,-0.000858270497959616));
#18761=CARTESIAN_POINT('Ctrl Pts',(10.5163317654776,-1.20384274018949,0.201614467507756));
#18762=CARTESIAN_POINT('Ctrl Pts',(10.5057293269973,-1.1932591813998,0.404087216090532));
#18763=CARTESIAN_POINT('Ctrl Pts',(10.4951269905998,-1.18267571840064,0.606559974437339));
#18764=CARTESIAN_POINT('Ctrl Pts',(10.5053655128635,-1.21565094114741,-0.0019246498908503));
#18765=CARTESIAN_POINT('Ctrl Pts',(10.4947646468921,-1.20506932615592,0.200548282383137));
#18766=CARTESIAN_POINT('Ctrl Pts',(10.4841638390504,-1.19448787589602,0.403021225840181));
#18767=CARTESIAN_POINT('Ctrl Pts',(10.4735630903435,-1.18390659316268,0.605494180667945));
#18768=CARTESIAN_POINT('Ctrl Pts',(10.5997255308004,-1.11583328740478,1.02782365951626E-16));
#18769=CARTESIAN_POINT('Ctrl Pts',(10.589152548365,-1.10529029582828,0.201744523047832));
#18770=CARTESIAN_POINT('Ctrl Pts',(10.5785795654695,-1.09474747266587,0.40348905487273));
#18771=CARTESIAN_POINT('Ctrl Pts',(10.5680065821063,-1.08420482079362,0.605233595624295));
#18772=CARTESIAN_POINT('Ctrl Pts',(10.5053638082297,1.21564923960921,-0.0018920919656423));
#18773=CARTESIAN_POINT('Ctrl Pts',(10.4947635104759,1.20506819181477,0.200569987667808));
#18774=CARTESIAN_POINT('Ctrl Pts',(10.4841632708454,1.19448730873444,0.403032078483127));
#18775=CARTESIAN_POINT('Ctrl Pts',(10.4735630903435,1.18390659316268,0.605494180667945));
#18776=CARTESIAN_POINT('Ctrl Pts',(10.5341220579192,1.21401666636749,-0.000470252816738081));
#18777=CARTESIAN_POINT('Ctrl Pts',(10.5235196325477,1.20343268662274,0.201991562854702));
#18778=CARTESIAN_POINT('Ctrl Pts',(10.5129172908767,1.19284910679518,0.404453403808947));
#18779=CARTESIAN_POINT('Ctrl Pts',(10.5023149573519,1.18226542681329,0.606915239027137));
#18780=CARTESIAN_POINT('Ctrl Pts',(10.5827170203615,1.18801090922716,0.000717463067903341));
#18781=CARTESIAN_POINT('Ctrl Pts',(10.5721088691741,1.17742555398174,0.203178921531494));
#18782=CARTESIAN_POINT('Ctrl Pts',(10.5615007184277,1.16684027916303,0.405640383775807));
#18783=CARTESIAN_POINT('Ctrl Pts',(10.5508925935528,1.15625520969485,0.60810185787831));
#18784=CARTESIAN_POINT('Ctrl Pts',(10.5997792798033,1.13754603572512,-0.00102559206997387));
#18785=CARTESIAN_POINT('Ctrl Pts',(10.5891686973038,1.12696411138589,0.201435946515793));
#18786=CARTESIAN_POINT('Ctrl Pts',(10.5785581831385,1.11638231376635,0.40389749513889));
#18787=CARTESIAN_POINT('Ctrl Pts',(10.5679475995174,1.10580071474959,0.606359050464716));
#18788=CARTESIAN_POINT('Ctrl Pts',(10.5998382764002,1.11594571320176,-0.00215131420076595));
#18789=CARTESIAN_POINT('Ctrl Pts',(10.5892277121014,1.10536524516024,0.200310313518148));
#18790=CARTESIAN_POINT('Ctrl Pts',(10.5786171473394,1.09478494672192,0.402771950076102));
#18791=CARTESIAN_POINT('Ctrl Pts',(10.5680065821063,1.08420482079361,0.605233595624295));
#18792=CARTESIAN_POINT('Ctrl Pts',(10.5680065821063,1.08420482079361,0.605233595624295));
#18793=CARTESIAN_POINT('Ctrl Pts',(10.5785795654695,1.09474747266587,0.40348905487273));
#18794=CARTESIAN_POINT('Ctrl Pts',(10.589152548365,1.10529029582828,0.201744523047831));
#18795=CARTESIAN_POINT('Ctrl Pts',(10.5997255308004,1.11583328740478,1.07661275727811E-16));
#18796=CARTESIAN_POINT('Ctrl Pts',(10.1947388861048,1.09885088260187,0.7));
#18797=CARTESIAN_POINT('Ctrl Pts',(10.285877616441,1.09404209584202,0.7));
#18798=CARTESIAN_POINT('Ctrl Pts',(10.3770124662346,1.0891584122264,0.7));
#18799=CARTESIAN_POINT('Ctrl Pts',(10.4681436286308,1.08420482079361,0.7));
#18800=CARTESIAN_POINT('Ctrl Pts',(10.196260416419,1.12768774893097,0.700000000000001));
#18801=CARTESIAN_POINT('Ctrl Pts',(10.2874149314686,1.12287675076168,0.699999949550842));
#18802=CARTESIAN_POINT('Ctrl Pts',(10.3785648662465,1.11799094453753,0.700000051218742));
#18803=CARTESIAN_POINT('Ctrl Pts',(10.4697107510168,1.11303515260326,0.7));
#18804=CARTESIAN_POINT('Ctrl Pts',(10.1988975981852,1.17766904563614,0.67669140632491));
#18805=CARTESIAN_POINT('Ctrl Pts',(10.2900793016129,1.17285439035486,0.676693724638983));
#18806=CARTESIAN_POINT('Ctrl Pts',(10.3812557252598,1.16796482352885,0.676696026813929));
#18807=CARTESIAN_POINT('Ctrl Pts',(10.4724269697127,1.16300539549315,0.676698381019544));
#18808=CARTESIAN_POINT('Ctrl Pts',(10.1999375452555,1.19737868557977,0.627098033786781));
#18809=CARTESIAN_POINT('Ctrl Pts',(10.2911301919381,1.19256517083271,0.627104033151799));
#18810=CARTESIAN_POINT('Ctrl Pts',(10.382317043787,1.18767684023183,0.627110048826767));
#18811=CARTESIAN_POINT('Ctrl Pts',(10.4734985149421,1.18271860027509,0.627116141711795));
#18812=CARTESIAN_POINT('Ctrl Pts',(10.1999999975038,1.19856231440453,0.605472757505366));
#18813=CARTESIAN_POINT('Ctrl Pts',(10.2911933328565,1.19375025772558,0.605479840815741));
#18814=CARTESIAN_POINT('Ctrl Pts',(10.3823809652617,1.18886335120032,0.605486986548286));
#18815=CARTESIAN_POINT('Ctrl Pts',(10.4735630903435,1.18390659316268,0.605494180667944));
#18816=CARTESIAN_POINT('Ctrl Pts',(0.200159601751749,1.12312829248604,-0.00219180147311912));
#18817=CARTESIAN_POINT('Ctrl Pts',(0.210770873167554,1.11255922017607,0.200283318842441));
#18818=CARTESIAN_POINT('Ctrl Pts',(0.221382145211419,1.10199037808008,0.402758451142111));
#18819=CARTESIAN_POINT('Ctrl Pts',(0.231993417893744,1.09142177001972,0.605233595624295));
#18820=CARTESIAN_POINT('Ctrl Pts',(0.200236952094631,1.15148086499205,-0.000715869007730825));
#18821=CARTESIAN_POINT('Ctrl Pts',(0.210848310847714,1.14090905181173,0.201759082033021));
#18822=CARTESIAN_POINT('Ctrl Pts',(0.221459381762758,1.13033759660317,0.404234066901971));
#18823=CARTESIAN_POINT('Ctrl Pts',(0.232070742664217,1.11976621744484,0.606709040139042));
#18824=CARTESIAN_POINT('Ctrl Pts',(0.222806696702742,1.20067708175657,0.000669311976984441));
#18825=CARTESIAN_POINT('Ctrl Pts',(0.233413416075889,1.19010082554658,0.203144236955742));
#18826=CARTESIAN_POINT('Ctrl Pts',(0.244020198555212,1.17952469009474,0.405619164345205));
#18827=CARTESIAN_POINT('Ctrl Pts',(0.254626870458834,1.16894881850735,0.608094110943904));
#18828=CARTESIAN_POINT('Ctrl Pts',(0.271086891015657,1.22096622390789,-0.000801865493577694));
#18829=CARTESIAN_POINT('Ctrl Pts',(0.281686280594249,1.21039315447922,0.201673594461172));
#18830=CARTESIAN_POINT('Ctrl Pts',(0.292285672737775,1.1998203699977,0.404149068703718));
#18831=CARTESIAN_POINT('Ctrl Pts',(0.302884933932915,1.18924771644243,0.606624555877912));
#18832=CARTESIAN_POINT('Ctrl Pts',(0.292287201081515,1.22267118699778,-0.00182392867695869));
#18833=CARTESIAN_POINT('Ctrl Pts',(0.302884364349574,1.21210098433295,0.200651796350731));
#18834=CARTESIAN_POINT('Ctrl Pts',(0.313481451159089,1.20153100270242,0.403127536304793));
#18835=CARTESIAN_POINT('Ctrl Pts',(0.324078460244491,1.19096124572524,0.605603291426262));
#18836=CARTESIAN_POINT('Origin',(10.6002740930491,1.4,-0.0104671912485891));
#18837=CARTESIAN_POINT('Origin',(0.331856371369202,1.09142177001972,0.6));
#18838=CARTESIAN_POINT('',(0.3318563713692,1.09142177001972,0.9));
#18839=CARTESIAN_POINT('',(0.0322675109428288,1.09142177001972,0.615700786872883));
#18840=CARTESIAN_POINT('Origin',(0.3318563713692,1.09142177001972,0.6));
#18841=CARTESIAN_POINT('',(0.308522637995069,1.39004019713626,0.616809874278785));
#18842=CARTESIAN_POINT('Origin',(0.331856371369202,1.09142177001972,0.6));
#18843=CARTESIAN_POINT('Origin',(0.331856371369201,1.09142177001972,0.6));
#18844=CARTESIAN_POINT('Origin',(10.4681436286308,1.08420482079361,0.6));
#18845=CARTESIAN_POINT('',(10.4681436286308,1.08420482109828,0.9));
#18846=CARTESIAN_POINT('',(10.4844020137689,1.3833101379008,0.616482542003833));
#18847=CARTESIAN_POINT('Origin',(10.4681436258201,1.08420482094639,0.6));
#18848=CARTESIAN_POINT('',(10.7677324890572,1.08420482079361,0.615700786872884));
#18849=CARTESIAN_POINT('Origin',(10.4681436286308,1.08420482079361,0.6));
#18850=CARTESIAN_POINT('Origin',(10.4681436286308,1.08420482079362,0.6));
#18851=CARTESIAN_POINT('Origin',(0.3318563713692,-1.09142177001972,0.6));
#18852=CARTESIAN_POINT('',(0.3318563713692,-1.09142177001972,0.9));
#18853=CARTESIAN_POINT('',(0.308522637995069,-1.39004019713626,0.616809874278785));
#18854=CARTESIAN_POINT('Origin',(0.3318563713692,-1.09142177001972,0.6));
#18855=CARTESIAN_POINT('',(0.0322675109428289,-1.09142177001972,0.615700786872884));
#18856=CARTESIAN_POINT('Origin',(0.3318563713692,-1.09142177001972,0.6));
#18857=CARTESIAN_POINT('Origin',(0.331856371369201,-1.09142177001972,0.6));
#18858=CARTESIAN_POINT('Origin',(0.3318563713692,-0.7,0.6));
#18859=CARTESIAN_POINT('',(0.0322675109428288,-0.7,0.615700786872883));
#18860=CARTESIAN_POINT('',(0.3318563713692,-0.7,0.9));
#18861=CARTESIAN_POINT('Ctrl Pts',(0.276048389810261,-1.42252533450788,
-0.00533608639730399));
#18862=CARTESIAN_POINT('Ctrl Pts',(0.28687338241706,-1.4116967417008,0.202045878554724));
#18863=CARTESIAN_POINT('Ctrl Pts',(0.297698133178874,-1.40086836142621,
0.409427865329919));
#18864=CARTESIAN_POINT('Ctrl Pts',(0.308522637995069,-1.39004019713626,
0.616809874278785));
#18865=CARTESIAN_POINT('Ctrl Pts',(0.191246496057484,-1.41570630783033,
-0.00124775669238285));
#18866=CARTESIAN_POINT('Ctrl Pts',(0.202080757839133,-1.40486573978029,
0.206133102090467));
#18867=CARTESIAN_POINT('Ctrl Pts',(0.212914648880055,-1.39402634701096,
0.413514041581016));
#18868=CARTESIAN_POINT('Ctrl Pts',(0.223748532748767,-1.38318608000504,
0.620894932085382));
#18869=CARTESIAN_POINT('Ctrl Pts',(0.0492682973509243,-1.33685850703924,
0.00207719607616587));
#18870=CARTESIAN_POINT('Ctrl Pts',(0.0601266125734448,-1.32601270457081,
0.209456583216085));
#18871=CARTESIAN_POINT('Ctrl Pts',(0.0709850253737815,-1.3151666447344,
0.416835949794532));
#18872=CARTESIAN_POINT('Ctrl Pts',(0.0818432319483421,-1.30432109509162,
0.624215353109623));
#18873=CARTESIAN_POINT('Ctrl Pts',(-0.000163444061205068,-1.18769013309795,
-0.00311869847265479));
#18874=CARTESIAN_POINT('Ctrl Pts',(0.0107049555364969,-1.17685886333949,
0.204261034729081));
#18875=CARTESIAN_POINT('Ctrl Pts',(0.0215730900970294,-1.16602762920277,
0.411640782964944));
#18876=CARTESIAN_POINT('Ctrl Pts',(0.0324414916763936,-1.15519677672624,
0.619020537031064));
#18877=CARTESIAN_POINT('Ctrl Pts',(-0.00033748371827097,-1.12389640457412,
-0.0064395729582146));
#18878=CARTESIAN_POINT('Ctrl Pts',(0.0105308471731094,-1.11307128361434,
0.200940534347673));
#18879=CARTESIAN_POINT('Ctrl Pts',(0.0213991787230862,-1.10224640406117,
0.408320654220332));
#18880=CARTESIAN_POINT('Ctrl Pts',(0.0322675109428289,-1.09142177001972,
0.615700786872884));
#18881=CARTESIAN_POINT('Ctrl Pts',(0.27632692456468,-1.42224670711126,5.13911829758129E-17));
#18882=CARTESIAN_POINT('Ctrl Pts',(0.287059068122268,-1.41151099373342,
0.20560326985903));
#18883=CARTESIAN_POINT('Ctrl Pts',(0.297790973931072,-1.40077548928706,
0.411206561171438));
#18884=CARTESIAN_POINT('Ctrl Pts',(0.308522637995069,-1.39004019713626,
0.616809874278785));
#18885=CARTESIAN_POINT('Ctrl Pts',(0.0322675109428289,-1.09142177001972,
0.615700786872884));
#18886=CARTESIAN_POINT('Ctrl Pts',(0.0215116733095221,-1.10213436178043,
0.410467178800746));
#18887=CARTESIAN_POINT('Ctrl Pts',(0.0107558363321879,-1.11284719399673,
0.205233583245308));
#18888=CARTESIAN_POINT('Ctrl Pts',(1.76901136968166E-16,-1.12356026268968,
-7.45931094670027E-17));
#18889=CARTESIAN_POINT('Origin',(10.4681436286308,-1.08420482109828,0.6));
#18890=CARTESIAN_POINT('',(10.7677324890572,-1.08420482079361,0.615700786872884));
#18891=CARTESIAN_POINT('',(10.4844020137689,-1.3833101379008,0.616482542003833));
#18892=CARTESIAN_POINT('Origin',(10.4681436286308,-1.08420482079361,0.600000000000001));
#18893=CARTESIAN_POINT('',(10.4681436258201,-1.08420482094639,0.9));
#18894=CARTESIAN_POINT('Origin',(10.4681436286308,-1.08420482109828,0.6));
#18895=CARTESIAN_POINT('Origin',(10.4681436286308,-1.08420482079361,0.6));
#18896=CARTESIAN_POINT('Origin',(10.4681436286308,0.7,0.6));
#18897=CARTESIAN_POINT('',(10.7677324890572,0.7,0.615700786872884));
#18898=CARTESIAN_POINT('',(10.4681436286308,0.7,0.9));
#18899=CARTESIAN_POINT('Ctrl Pts',(10.4681436286308,-1.08420482079361,0.9));
#18900=CARTESIAN_POINT('Ctrl Pts',(9.02115959826777,-1.16285813221549,0.9));
#18901=CARTESIAN_POINT('Ctrl Pts',(5.64262097844114,-1.30550334054488,0.9));
#18902=CARTESIAN_POINT('Ctrl Pts',(2.25816172369615,-1.24194126716656,0.9));
#18903=CARTESIAN_POINT('Ctrl Pts',(0.331856371369198,-1.09142177001972,
0.9));
#18904=CARTESIAN_POINT('Ctrl Pts',(10.4728449957889,-1.17069581622255,0.9));
#18905=CARTESIAN_POINT('Ctrl Pts',(9.02515960257209,-1.24945398332951,0.900002463983243));
#18906=CARTESIAN_POINT('Ctrl Pts',(5.64406008560805,-1.39235654229312,0.899995181674544));
#18907=CARTESIAN_POINT('Ctrl Pts',(2.25481214769604,-1.3286896492945,0.900006992415263));
#18908=CARTESIAN_POINT('Ctrl Pts',(0.325113511056834,-1.17771496230318,
0.9));
#18909=CARTESIAN_POINT('Ctrl Pts',(10.4809942371438,-1.32061731204901,0.830050158657121));
#18910=CARTESIAN_POINT('Ctrl Pts',(9.03210079995546,-1.3995487214628,0.829938185878055));
#18911=CARTESIAN_POINT('Ctrl Pts',(5.64656962219688,-1.54290142969263,0.82970437227026));
#18912=CARTESIAN_POINT('Ctrl Pts',(2.24896854757963,-1.47903552984056,0.829838703712927));
#18913=CARTESIAN_POINT('Ctrl Pts',(0.313425270489114,-1.32729771265557,
0.830156825336737));
#18914=CARTESIAN_POINT('Ctrl Pts',(10.4842082875648,-1.37974615923803,0.681348425135383));
#18915=CARTESIAN_POINT('Ctrl Pts',(9.03482793853036,-1.45862084618981,0.681058092399338));
#18916=CARTESIAN_POINT('Ctrl Pts',(5.64753778607331,-1.60187726023264,0.68045297450285));
#18917=CARTESIAN_POINT('Ctrl Pts',(2.24670449952385,-1.53809938127555,0.680799765935021));
#18918=CARTESIAN_POINT('Ctrl Pts',(0.308806004580392,-1.38641375285276,
0.681625057916928));
#18919=CARTESIAN_POINT('Ctrl Pts',(10.4844020137689,-1.3833101379008,0.616482542003833));
#18920=CARTESIAN_POINT('Ctrl Pts',(9.03499042108131,-1.46211428773623,0.616139856494792));
#18921=CARTESIAN_POINT('Ctrl Pts',(5.64759185703765,-1.60522711936681,0.615422163720642));
#18922=CARTESIAN_POINT('Ctrl Pts',(2.24657199659733,-1.54153220865049,0.615835494619844));
#18923=CARTESIAN_POINT('Ctrl Pts',(0.308522637995066,-1.39004019713626,
0.616809874278785));
#18924=CARTESIAN_POINT('Ctrl Pts',(0.308522637995066,-1.39004019713626,
0.616809874278785));
#18925=CARTESIAN_POINT('Ctrl Pts',(2.24657199659733,-1.54153220865049,0.615835494619844));
#18926=CARTESIAN_POINT('Ctrl Pts',(5.64759185703765,-1.60522711936681,0.615422163720642));
#18927=CARTESIAN_POINT('Ctrl Pts',(9.03499042108131,-1.46211428773623,0.616139856494792));
#18928=CARTESIAN_POINT('Ctrl Pts',(10.4844020137689,-1.3833101379008,0.616482542003833));
#18929=CARTESIAN_POINT('Ctrl Pts',(10.4681436258201,-1.08420482094639,0.900000000000001));
#18930=CARTESIAN_POINT('Ctrl Pts',(9.02115959639274,-1.16285813229465,0.9));
#18931=CARTESIAN_POINT('Ctrl Pts',(5.64262097750198,-1.30550334052724,0.9));
#18932=CARTESIAN_POINT('Ctrl Pts',(2.25816172369615,-1.24194126716656,0.9));
#18933=CARTESIAN_POINT('Ctrl Pts',(0.331856371369198,-1.09142177001972,
0.9));
#18934=CARTESIAN_POINT('Ctrl Pts',(10.8003433549902,-1.11672267507076,-0.00655160349952438));
#18935=CARTESIAN_POINT('Ctrl Pts',(10.7894730668347,-1.10588321133639,0.200865850630566));
#18936=CARTESIAN_POINT('Ctrl Pts',(10.7786027781932,-1.09504392553578,0.408283314033857));
#18937=CARTESIAN_POINT('Ctrl Pts',(10.7677324890572,-1.08420482079361,0.615700786872885));
#18938=CARTESIAN_POINT('Ctrl Pts',(10.8001073672393,-1.20312439623403,-0.00204868896805508));
#18939=CARTESIAN_POINT('Ctrl Pts',(10.7892368724076,-1.19227880391739,0.205368384315645));
#18940=CARTESIAN_POINT('Ctrl Pts',(10.7783670568079,-1.18143370221047,0.41278551899075));
#18941=CARTESIAN_POINT('Ctrl Pts',(10.7674965587017,-1.17058839661753,0.620202606234566));
#18942=CARTESIAN_POINT('Ctrl Pts',(10.7300137544668,-1.35289768637741,0.00210488808650419));
#18943=CARTESIAN_POINT('Ctrl Pts',(10.7191538066016,-1.34204221082848,0.209521911971666));
#18944=CARTESIAN_POINT('Ctrl Pts',(10.7082938463195,-1.33118673671862,0.416938933985702));
#18945=CARTESIAN_POINT('Ctrl Pts',(10.6974340169938,-1.32033143065575,0.624355970618915));
#18946=CARTESIAN_POINT('Ctrl Pts',(10.5816241002662,-1.4121605627967,-0.00257485550010117));
#18947=CARTESIAN_POINT('Ctrl Pts',(10.5707805459565,-1.4013126969686,0.204843391064434));
#18948=CARTESIAN_POINT('Ctrl Pts',(10.5599369567012,-1.39046512672587,0.412261650129749));
#18949=CARTESIAN_POINT('Ctrl Pts',(10.5490937145378,-1.37961751361469,0.619679923312015));
#18950=CARTESIAN_POINT('Ctrl Pts',(10.5169176890673,-1.41583338198674,-0.00577403633861717));
#18951=CARTESIAN_POINT('Ctrl Pts',(10.5060789456421,-1.40499213715574,0.201644806368331));
#18952=CARTESIAN_POINT('Ctrl Pts',(10.4952403861233,-1.39415105487295,0.40906366572247));
#18953=CARTESIAN_POINT('Ctrl Pts',(10.4844020137689,-1.3833101379008,0.616482542003833));
#18954=CARTESIAN_POINT('Ctrl Pts',(10.8,-1.11638029377732,-2.51534904016637E-17));
#18955=CARTESIAN_POINT('Ctrl Pts',(10.7892441634977,-1.10565496086826,0.205233586491178));
#18956=CARTESIAN_POINT('Ctrl Pts',(10.7784883265195,-1.09492980219801,0.410467182062988));
#18957=CARTESIAN_POINT('Ctrl Pts',(10.7677324890572,-1.08420482079361,0.615700786872885));
#18958=CARTESIAN_POINT('Ctrl Pts',(10.4844020137689,-1.3833101379008,0.616482542003833));
#18959=CARTESIAN_POINT('Ctrl Pts',(10.4951398148107,-1.39405045994841,0.410988344812119));
#18960=CARTESIAN_POINT('Ctrl Pts',(10.5058777995597,-1.40479094425298,0.205494164234945));
#18961=CARTESIAN_POINT('Ctrl Pts',(10.5166159648474,-1.4155315881283,-2.5652223401007E-16));
#18962=CARTESIAN_POINT('Ctrl Pts',(10.5169125872774,1.41582827901939,-0.0056764044152427));
#18963=CARTESIAN_POINT('Ctrl Pts',(10.5060755445066,1.40498873522851,0.20170989432247));
#18964=CARTESIAN_POINT('Ctrl Pts',(10.4952386855848,1.39414935393528,0.409096209702196));
#18965=CARTESIAN_POINT('Ctrl Pts',(10.4844020137689,1.3833101379008,0.616482542003833));
#18966=CARTESIAN_POINT('Ctrl Pts',(10.6031877991504,1.41093118264609,-0.00141083033817288));
#18967=CARTESIAN_POINT('Ctrl Pts',(10.5923442181457,1.40008262840665,0.205974657203891));
#18968=CARTESIAN_POINT('Ctrl Pts',(10.5815009048179,1.38923496752292,0.413360205434192));
#18969=CARTESIAN_POINT('Ctrl Pts',(10.5706576147941,1.37838663885266,0.62074571708141));
#18970=CARTESIAN_POINT('Ctrl Pts',(10.7489822201969,1.33286898269122,0.00215046584238339));
#18971=CARTESIAN_POINT('Ctrl Pts',(10.7381210493968,1.32201618867047,0.209534855263179));
#18972=CARTESIAN_POINT('Ctrl Pts',(10.7272598662103,1.31116338896628,0.416919242515175));
#18973=CARTESIAN_POINT('Ctrl Pts',(10.716398780155,1.30031077634578,0.624303643734563));
#18974=CARTESIAN_POINT('Ctrl Pts',(10.8001612475457,1.18151886169146,-0.00307678645922502));
#18975=CARTESIAN_POINT('Ctrl Pts',(10.7892926103682,1.17067663552019,0.20430785074418));
#18976=CARTESIAN_POINT('Ctrl Pts',(10.7784241800195,1.15983442267521,0.41169249890798));
#18977=CARTESIAN_POINT('Ctrl Pts',(10.7675555412906,1.14899250266155,0.619077151394146));
#18978=CARTESIAN_POINT('Ctrl Pts',(10.8003382383521,1.11671757294177,-0.00645397222975308));
#18979=CARTESIAN_POINT('Ctrl Pts',(10.7894696557425,1.1058798099729,0.200930938146656));
#18980=CARTESIAN_POINT('Ctrl Pts',(10.778601072647,1.09504222488243,0.408315857793383));
#18981=CARTESIAN_POINT('Ctrl Pts',(10.7677324890572,1.08420482079361,0.615700786872884));
#18982=CARTESIAN_POINT('Ctrl Pts',(10.5166159648474,1.4155315881283,3.37837396946483E-16));
#18983=CARTESIAN_POINT('Ctrl Pts',(10.5058777995597,1.40479094425298,0.205494164234944));
#18984=CARTESIAN_POINT('Ctrl Pts',(10.4951398148107,1.39405045994841,0.41098834481212));
#18985=CARTESIAN_POINT('Ctrl Pts',(10.4844020137689,1.3833101379008,0.616482542003833));
#18986=CARTESIAN_POINT('Ctrl Pts',(10.7677324890572,1.08420482079361,0.615700786872884));
#18987=CARTESIAN_POINT('Ctrl Pts',(10.7784883265195,1.09492980219801,0.410467182062988));
#18988=CARTESIAN_POINT('Ctrl Pts',(10.7892441634977,1.10565496086826,0.205233586491177));
#18989=CARTESIAN_POINT('Ctrl Pts',(10.8,1.11638029377732,-4.7271214720368E-17));
#18990=CARTESIAN_POINT('Ctrl Pts',(0.3318563713692,1.09142177001972,0.9));
#18991=CARTESIAN_POINT('Ctrl Pts',(1.77658538561441,1.20431139287985,0.9));
#18992=CARTESIAN_POINT('Ctrl Pts',(5.15852145577913,1.31798734362749,0.900000000000001));
#18993=CARTESIAN_POINT('Ctrl Pts',(8.53883158814675,1.18907590268945,0.9));
#18994=CARTESIAN_POINT('Ctrl Pts',(10.4681436286308,1.08420482079361,0.9));
#18995=CARTESIAN_POINT('Ctrl Pts',(0.325113511056836,1.17771496230318,0.9));
#18996=CARTESIAN_POINT('Ctrl Pts',(1.77238748853623,1.29094597754667,0.900005244311447));
#18997=CARTESIAN_POINT('Ctrl Pts',(5.15940689953628,1.40489117512763,0.899995532233175));
#18998=CARTESIAN_POINT('Ctrl Pts',(8.54259780483314,1.2757067056985,0.90000328531099));
#18999=CARTESIAN_POINT('Ctrl Pts',(10.4728449957889,1.17069581622255,0.9));
#19000=CARTESIAN_POINT('Ctrl Pts',(0.313425270489116,1.32729771265557,0.830156825336737));
#19001=CARTESIAN_POINT('Ctrl Pts',(1.76508272830699,1.44110107554431,0.829918234118879));
#19002=CARTESIAN_POINT('Ctrl Pts',(5.16095094050242,1.55552201031752,0.829677185710002));
#19003=CARTESIAN_POINT('Ctrl Pts',(8.54913632089268,1.4258591912674,0.829900861618366));
#19004=CARTESIAN_POINT('Ctrl Pts',(10.4809942371438,1.32061731204901,0.830050158657121));
#19005=CARTESIAN_POINT('Ctrl Pts',(0.308806004580394,1.38641375285276,0.681625057916928));
#19006=CARTESIAN_POINT('Ctrl Pts',(1.76222987578798,1.50017797416985,0.681006088930498));
#19007=CARTESIAN_POINT('Ctrl Pts',(5.16154986224672,1.61450132085358,0.68038246417749));
#19008=CARTESIAN_POINT('Ctrl Pts',(8.55170115551887,1.48491240850707,0.680961314820656));
#19009=CARTESIAN_POINT('Ctrl Pts',(10.4842082875648,1.37974615923803,0.681348425135383));
#19010=CARTESIAN_POINT('Ctrl Pts',(0.308522637995068,1.39004019713626,0.616809874278785));
#19011=CARTESIAN_POINT('Ctrl Pts',(1.76205965694675,1.50365920577193,0.616079089534579));
#19012=CARTESIAN_POINT('Ctrl Pts',(5.16158497046229,1.61783515152865,0.615338844765104));
#19013=CARTESIAN_POINT('Ctrl Pts',(8.55185322351876,1.48838233768137,0.616025627991778));
#19014=CARTESIAN_POINT('Ctrl Pts',(10.4844020137689,1.3833101379008,0.616482542003833));
#19015=CARTESIAN_POINT('Ctrl Pts',(10.4844020137689,1.3833101379008,0.616482542003833));
#19016=CARTESIAN_POINT('Ctrl Pts',(8.55185322351876,1.48838233768137,0.616025627991778));
#19017=CARTESIAN_POINT('Ctrl Pts',(5.16158497046229,1.61783515152865,0.615338844765104));
#19018=CARTESIAN_POINT('Ctrl Pts',(1.76205965694675,1.50365920577193,0.616079089534579));
#19019=CARTESIAN_POINT('Ctrl Pts',(0.308522637995068,1.39004019713626,0.616809874278785));
#19020=CARTESIAN_POINT('Ctrl Pts',(0.3318563713692,1.09142177001972,0.9));
#19021=CARTESIAN_POINT('Ctrl Pts',(1.77658538561441,1.20431139287985,0.9));
#19022=CARTESIAN_POINT('Ctrl Pts',(5.15852145577913,1.31798734362749,0.900000000000001));
#19023=CARTESIAN_POINT('Ctrl Pts',(8.53883158814675,1.18907590268945,0.9));
#19024=CARTESIAN_POINT('Ctrl Pts',(10.4681436286308,1.08420482079361,0.9));
#19025=CARTESIAN_POINT('Ctrl Pts',(-0.000344602063817145,1.12390349461883,
-0.00657539908256866));
#19026=CARTESIAN_POINT('Ctrl Pts',(0.0105261016091243,1.11307601020539,
0.200849983592616));
#19027=CARTESIAN_POINT('Ctrl Pts',(0.0213968059409475,1.10224876730309,
0.408275378840013));
#19028=CARTESIAN_POINT('Ctrl Pts',(0.0322675109428289,1.09142177001972,
0.615700786872884));
#19029=CARTESIAN_POINT('Ctrl Pts',(-0.000112549170678945,1.2089618047365,
-0.00214756610981592));
#19030=CARTESIAN_POINT('Ctrl Pts',(0.0107584275574203,1.19812589474889,
0.205277296000037));
#19031=CARTESIAN_POINT('Ctrl Pts',(0.021628504370896,1.18729063034778,0.412702239156743));
#19032=CARTESIAN_POINT('Ctrl Pts',(0.0324994852542487,1.17645511229507,
0.620127120417125));
#19033=CARTESIAN_POINT('Ctrl Pts',(0.0675181008536004,1.35659180908255,
0.00201426213057289));
#19034=CARTESIAN_POINT('Ctrl Pts',(0.0783748317004002,1.34574224493831,
0.20943904356877));
#19035=CARTESIAN_POINT('Ctrl Pts',(0.0892318011706237,1.33489254525337,
0.416863803530356));
#19036=CARTESIAN_POINT('Ctrl Pts',(0.100088380073201,1.32404321751407,0.624288602298589));
#19037=CARTESIAN_POINT('Ctrl Pts',(0.212439875011655,1.41741816253371,-0.00240566592686199));
#19038=CARTESIAN_POINT('Ctrl Pts',(0.223274062163905,1.40657840226088,0.20502076110302));
#19039=CARTESIAN_POINT('Ctrl Pts',(0.234108278795672,1.39573903465802,0.412447205628077));
#19040=CARTESIAN_POINT('Ctrl Pts',(0.244942059060342,1.38489960928785,0.619873667633733));
#19041=CARTESIAN_POINT('Ctrl Pts',(0.276041299849618,1.42253242682652,-0.00547191373834488));
#19042=CARTESIAN_POINT('Ctrl Pts',(0.286868655882245,1.41170146982041,0.201955326984501));
#19043=CARTESIAN_POINT('Ctrl Pts',(0.297695769965166,1.40087072543886,0.409382589539965));
#19044=CARTESIAN_POINT('Ctrl Pts',(0.308522637995069,1.39004019713626,0.616809874278785));
#19045=CARTESIAN_POINT('Ctrl Pts',(2.26869304592592E-17,1.12356026268968,
-3.16587034365767E-17));
#19046=CARTESIAN_POINT('Ctrl Pts',(0.0107558363321878,1.11284719399672,
0.205233583245308));
#19047=CARTESIAN_POINT('Ctrl Pts',(0.0215116733095221,1.10213436178043,
0.410467178800746));
#19048=CARTESIAN_POINT('Ctrl Pts',(0.0322675109428289,1.09142177001972,
0.615700786872884));
#19049=CARTESIAN_POINT('Ctrl Pts',(0.308522637995069,1.39004019713626,0.616809874278785));
#19050=CARTESIAN_POINT('Ctrl Pts',(0.297790973931072,1.40077548928706,0.411206561171438));
#19051=CARTESIAN_POINT('Ctrl Pts',(0.287059068122271,1.41151099373341,0.205603269859031));
#19052=CARTESIAN_POINT('Ctrl Pts',(0.276326924564681,1.42224670711126,-2.68882138776405E-16));
#19053=CARTESIAN_POINT('Ctrl Pts',(10.5166159648474,-1.4155315881283,0.));
#19054=CARTESIAN_POINT('Ctrl Pts',(10.5064062201588,-1.40475637621136,0.205603291426271));
#19055=CARTESIAN_POINT('Ctrl Pts',(10.4961964754701,-1.39398116429443,0.411206582852543));
#19056=CARTESIAN_POINT('Ctrl Pts',(10.4859867307814,-1.38320595237749,0.616809874278814));
#19057=CARTESIAN_POINT('Ctrl Pts',(7.10318628475318,-1.599994843061,0.));
#19058=CARTESIAN_POINT('Ctrl Pts',(7.09978773046573,-1.58921963114407,0.205603291426271));
#19059=CARTESIAN_POINT('Ctrl Pts',(7.09638917617828,-1.57844441922713,0.411206582852543));
#19060=CARTESIAN_POINT('Ctrl Pts',(7.09299062189083,-1.5676692073102,0.616809874278814));
#19061=CARTESIAN_POINT('Ctrl Pts',(3.68975660465893,-1.68747752195839,0.));
#19062=CARTESIAN_POINT('Ctrl Pts',(3.69316924077269,-1.67670231004145,0.205603291426272));
#19063=CARTESIAN_POINT('Ctrl Pts',(3.69658187688646,-1.66592709812452,0.411206582852543));
#19064=CARTESIAN_POINT('Ctrl Pts',(3.69999451300023,-1.65515188620758,0.616809874278814));
#19065=CARTESIAN_POINT('Ctrl Pts',(0.276326924564679,-1.42224670711126,
0.));
#19066=CARTESIAN_POINT('Ctrl Pts',(0.286550751079662,-1.41147149519433,
0.205603291426271));
#19067=CARTESIAN_POINT('Ctrl Pts',(0.296774577594646,-1.40069628327739,
0.411206582852543));
#19068=CARTESIAN_POINT('Ctrl Pts',(0.306998404109629,-1.38992107136046,
0.616809874278814));
#19069=CARTESIAN_POINT('Origin',(0.,-1.4,0.));
#19070=CARTESIAN_POINT('Origin',(5.4,-8.13935059369636E-18,0.9));
#19071=CARTESIAN_POINT('Ctrl Pts',(0.276326924564679,1.42224670711126,0.));
#19072=CARTESIAN_POINT('Ctrl Pts',(0.286550751079662,1.41147149519433,0.205603291426271));
#19073=CARTESIAN_POINT('Ctrl Pts',(0.296774577594645,1.40069628327739,0.411206582852543));
#19074=CARTESIAN_POINT('Ctrl Pts',(0.306998404109628,1.38992107136046,0.616809874278814));
#19075=CARTESIAN_POINT('Ctrl Pts',(3.68975660465893,1.68747752195839,0.));
#19076=CARTESIAN_POINT('Ctrl Pts',(3.6931692407727,1.67670231004145,0.205603291426271));
#19077=CARTESIAN_POINT('Ctrl Pts',(3.69658187688646,1.66592709812452,0.411206582852543));
#19078=CARTESIAN_POINT('Ctrl Pts',(3.69999451300023,1.65515188620758,0.616809874278814));
#19079=CARTESIAN_POINT('Ctrl Pts',(7.10318628475318,1.599994843061,0.));
#19080=CARTESIAN_POINT('Ctrl Pts',(7.09978773046573,1.58921963114407,0.205603291426271));
#19081=CARTESIAN_POINT('Ctrl Pts',(7.09638917617828,1.57844441922713,0.411206582852543));
#19082=CARTESIAN_POINT('Ctrl Pts',(7.09299062189083,1.5676692073102,0.616809874278814));
#19083=CARTESIAN_POINT('Ctrl Pts',(10.5166159648474,1.4155315881283,0.));
#19084=CARTESIAN_POINT('Ctrl Pts',(10.5064062201588,1.40475637621136,0.205603291426271));
#19085=CARTESIAN_POINT('Ctrl Pts',(10.4961964754701,1.39398116429443,0.411206582852543));
#19086=CARTESIAN_POINT('Ctrl Pts',(10.4859867307814,1.38320595237749,0.616809874278814));
#19087=CARTESIAN_POINT('Origin',(10.8,1.4,0.));
#24791=UNCERTAINTY_MEASURE_WITH_UNIT(LENGTH_MEASURE(0.001),#24810,
'DISTANCE_ACCURACY_VALUE',
'Maximum model space distance between geometric entities at asserted c
onnectivities');
#24796=UNCERTAINTY_MEASURE_WITH_UNIT(LENGTH_MEASURE(0.001),#24810,
'DISTANCE_ACCURACY_VALUE',
'Maximum model space distance between geometric entities at asserted c
onnectivities');
#24804=(
GEOMETRIC_REPRESENTATION_CONTEXT(3)
GLOBAL_UNCERTAINTY_ASSIGNED_CONTEXT((#24791))
GLOBAL_UNIT_ASSIGNED_CONTEXT((#24810,#24812,#24813))
REPRESENTATION_CONTEXT('','3D')
);
#24809=(
GEOMETRIC_REPRESENTATION_CONTEXT(3)
GLOBAL_UNCERTAINTY_ASSIGNED_CONTEXT((#24796))
GLOBAL_UNIT_ASSIGNED_CONTEXT((#24810,#24812,#24813))
REPRESENTATION_CONTEXT('','3D')
);
#24810=(
LENGTH_UNIT()
NAMED_UNIT(*)
SI_UNIT(.CENTI.,.METRE.)
);
#24812=(
NAMED_UNIT(*)
PLANE_ANGLE_UNIT()
SI_UNIT($,.RADIAN.)
);
#24813=(
NAMED_UNIT(*)
SI_UNIT($,.STERADIAN.)
SOLID_ANGLE_UNIT()
);
#24821=SHAPE_DEFINITION_REPRESENTATION(#24833,#24861);
#24833=PRODUCT_DEFINITION_SHAPE('',$,#24874);
#24861=SHAPE_REPRESENTATION('',(#10371),#24804);
#24866=PRODUCT_DEFINITION_CONTEXT('part definition',#24904,'design');
#24874=PRODUCT_DEFINITION('2026-11-10-05-11-11-298',
'Lower structural shell',#24886,#24866);
#24886=PRODUCT_DEFINITION_FORMATION('',$,#24913);
#24904=APPLICATION_CONTEXT(
'Core Data for Automotive Mechanical Design Process');
#24905=PRODUCT_CONTEXT('part definition',#24904,'mechanical');
#24913=PRODUCT('2026-11-10-05-11-11-298','Lower structural shell',$,(#24905));
#24922=PRESENTATION_STYLE_ASSIGNMENT((#24930));
#24930=SURFACE_STYLE_USAGE(.BOTH.,#24938);
#24938=SURFACE_SIDE_STYLE('',(#24946));
#24946=SURFACE_STYLE_FILL_AREA(#24954);
#24954=FILL_AREA_STYLE('Structural dark blue',(#24962));
#24962=FILL_AREA_STYLE_COLOUR('Structural dark blue',#24970);
#24970=COLOUR_RGB('Structural dark blue',0.0901960784313725,0.270588235294118,
0.513725490196078);
ENDSEC;
END-ISO-10303-21;
